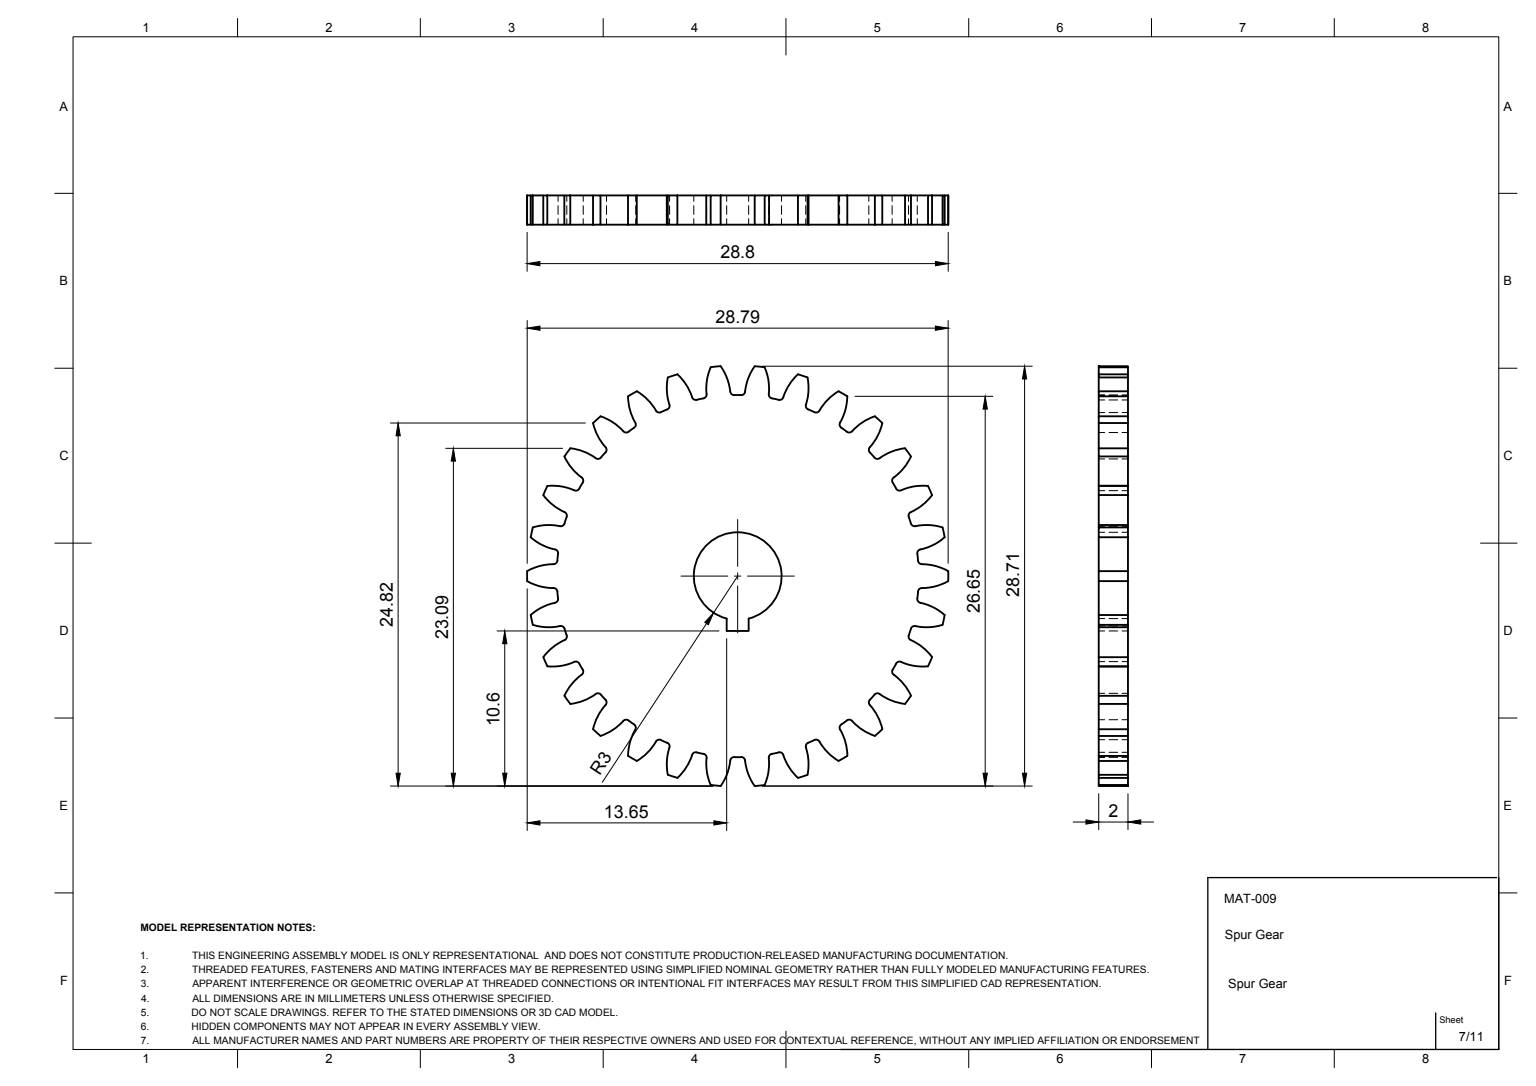
ISO-10303-21;
HEADER;
/* Generated by software containing ST-Developer
 * from STEP Tools, Inc. (www.steptools.com) 
 */

FILE_DESCRIPTION(
/* description */ ('STEP AP214'),
/* implementation_level */ '2;1');

FILE_NAME(
/* name */ 'Spur Gear.step',
/* time_stamp */ '2026-11-14T05:43:09-08:00',
/* author */ (''),
/* organization */ (''),
/* preprocessor_version */ 'ST-DEVELOPER v20.2',
/* originating_system */ 'Autodesk Translation Framework v15.17.0.0',
/* authorisation */ '');

FILE_SCHEMA (('AUTOMOTIVE_DESIGN { 1 0 10303 214 3 1 1 }'));
ENDSEC;

DATA;
#10=MECHANICAL_DESIGN_GEOMETRIC_PRESENTATION_REPRESENTATION('',(#149),#11933);
#131=SHAPE_REPRESENTATION_RELATIONSHIP('SRR','None',#11991,#140);
#140=ADVANCED_BREP_SHAPE_REPRESENTATION('',(#158),#11927);
#149=STYLED_ITEM('',(#12043),#158);
#158=MANIFOLD_SOLID_BREP('Body1',#6646);
#192=FACE_BOUND('',#825,.T.);
#193=FACE_BOUND('',#827,.T.);
#251=PLANE('',#7044);
#252=PLANE('',#7178);
#253=PLANE('',#7445);
#254=PLANE('',#7446);
#255=PLANE('',#7447);
#394=FACE_OUTER_BOUND('',#776,.T.);
#395=FACE_OUTER_BOUND('',#777,.T.);
#396=FACE_OUTER_BOUND('',#778,.T.);
#397=FACE_OUTER_BOUND('',#779,.T.);
#398=FACE_OUTER_BOUND('',#780,.T.);
#399=FACE_OUTER_BOUND('',#781,.T.);
#400=FACE_OUTER_BOUND('',#782,.T.);
#401=FACE_OUTER_BOUND('',#783,.T.);
#402=FACE_OUTER_BOUND('',#784,.T.);
#403=FACE_OUTER_BOUND('',#785,.T.);
#404=FACE_OUTER_BOUND('',#786,.T.);
#405=FACE_OUTER_BOUND('',#787,.T.);
#406=FACE_OUTER_BOUND('',#788,.T.);
#407=FACE_OUTER_BOUND('',#789,.T.);
#408=FACE_OUTER_BOUND('',#790,.T.);
#409=FACE_OUTER_BOUND('',#791,.T.);
#410=FACE_OUTER_BOUND('',#792,.T.);
#411=FACE_OUTER_BOUND('',#793,.T.);
#412=FACE_OUTER_BOUND('',#794,.T.);
#413=FACE_OUTER_BOUND('',#795,.T.);
#414=FACE_OUTER_BOUND('',#796,.T.);
#415=FACE_OUTER_BOUND('',#797,.T.);
#416=FACE_OUTER_BOUND('',#798,.T.);
#417=FACE_OUTER_BOUND('',#799,.T.);
#418=FACE_OUTER_BOUND('',#800,.T.);
#419=FACE_OUTER_BOUND('',#801,.T.);
#420=FACE_OUTER_BOUND('',#802,.T.);
#421=FACE_OUTER_BOUND('',#803,.T.);
#422=FACE_OUTER_BOUND('',#804,.T.);
#423=FACE_OUTER_BOUND('',#805,.T.);
#424=FACE_OUTER_BOUND('',#806,.T.);
#425=FACE_OUTER_BOUND('',#807,.T.);
#426=FACE_OUTER_BOUND('',#808,.T.);
#427=FACE_OUTER_BOUND('',#809,.T.);
#428=FACE_OUTER_BOUND('',#810,.T.);
#429=FACE_OUTER_BOUND('',#811,.T.);
#430=FACE_OUTER_BOUND('',#812,.T.);
#431=FACE_OUTER_BOUND('',#813,.T.);
#432=FACE_OUTER_BOUND('',#814,.T.);
#433=FACE_OUTER_BOUND('',#815,.T.);
#434=FACE_OUTER_BOUND('',#816,.T.);
#435=FACE_OUTER_BOUND('',#817,.T.);
#436=FACE_OUTER_BOUND('',#818,.T.);
#437=FACE_OUTER_BOUND('',#819,.T.);
#438=FACE_OUTER_BOUND('',#820,.T.);
#439=FACE_OUTER_BOUND('',#821,.T.);
#440=FACE_OUTER_BOUND('',#822,.T.);
#441=FACE_OUTER_BOUND('',#823,.T.);
#442=FACE_OUTER_BOUND('',#824,.T.);
#443=FACE_OUTER_BOUND('',#826,.T.);
#444=FACE_OUTER_BOUND('',#828,.T.);
#445=FACE_OUTER_BOUND('',#829,.T.);
#446=FACE_OUTER_BOUND('',#830,.T.);
#447=FACE_OUTER_BOUND('',#831,.T.);
#448=FACE_OUTER_BOUND('',#832,.T.);
#449=FACE_OUTER_BOUND('',#833,.T.);
#450=FACE_OUTER_BOUND('',#834,.T.);
#451=FACE_OUTER_BOUND('',#835,.T.);
#452=FACE_OUTER_BOUND('',#836,.T.);
#453=FACE_OUTER_BOUND('',#837,.T.);
#454=FACE_OUTER_BOUND('',#838,.T.);
#455=FACE_OUTER_BOUND('',#839,.T.);
#456=FACE_OUTER_BOUND('',#840,.T.);
#457=FACE_OUTER_BOUND('',#841,.T.);
#458=FACE_OUTER_BOUND('',#842,.T.);
#459=FACE_OUTER_BOUND('',#843,.T.);
#460=FACE_OUTER_BOUND('',#844,.T.);
#461=FACE_OUTER_BOUND('',#845,.T.);
#462=FACE_OUTER_BOUND('',#846,.T.);
#463=FACE_OUTER_BOUND('',#847,.T.);
#464=FACE_OUTER_BOUND('',#848,.T.);
#465=FACE_OUTER_BOUND('',#849,.T.);
#466=FACE_OUTER_BOUND('',#850,.T.);
#467=FACE_OUTER_BOUND('',#851,.T.);
#468=FACE_OUTER_BOUND('',#852,.T.);
#469=FACE_OUTER_BOUND('',#853,.T.);
#470=FACE_OUTER_BOUND('',#854,.T.);
#471=FACE_OUTER_BOUND('',#855,.T.);
#472=FACE_OUTER_BOUND('',#856,.T.);
#473=FACE_OUTER_BOUND('',#857,.T.);
#474=FACE_OUTER_BOUND('',#858,.T.);
#475=FACE_OUTER_BOUND('',#859,.T.);
#476=FACE_OUTER_BOUND('',#860,.T.);
#477=FACE_OUTER_BOUND('',#861,.T.);
#478=FACE_OUTER_BOUND('',#862,.T.);
#479=FACE_OUTER_BOUND('',#863,.T.);
#480=FACE_OUTER_BOUND('',#864,.T.);
#481=FACE_OUTER_BOUND('',#865,.T.);
#482=FACE_OUTER_BOUND('',#866,.T.);
#483=FACE_OUTER_BOUND('',#867,.T.);
#484=FACE_OUTER_BOUND('',#868,.T.);
#485=FACE_OUTER_BOUND('',#869,.T.);
#486=FACE_OUTER_BOUND('',#870,.T.);
#487=FACE_OUTER_BOUND('',#871,.T.);
#488=FACE_OUTER_BOUND('',#872,.T.);
#489=FACE_OUTER_BOUND('',#873,.T.);
#490=FACE_OUTER_BOUND('',#874,.T.);
#491=FACE_OUTER_BOUND('',#875,.T.);
#492=FACE_OUTER_BOUND('',#876,.T.);
#493=FACE_OUTER_BOUND('',#877,.T.);
#494=FACE_OUTER_BOUND('',#878,.T.);
#495=FACE_OUTER_BOUND('',#879,.T.);
#496=FACE_OUTER_BOUND('',#880,.T.);
#497=FACE_OUTER_BOUND('',#881,.T.);
#498=FACE_OUTER_BOUND('',#882,.T.);
#499=FACE_OUTER_BOUND('',#883,.T.);
#500=FACE_OUTER_BOUND('',#884,.T.);
#501=FACE_OUTER_BOUND('',#885,.T.);
#502=FACE_OUTER_BOUND('',#886,.T.);
#503=FACE_OUTER_BOUND('',#887,.T.);
#504=FACE_OUTER_BOUND('',#888,.T.);
#505=FACE_OUTER_BOUND('',#889,.T.);
#506=FACE_OUTER_BOUND('',#890,.T.);
#507=FACE_OUTER_BOUND('',#891,.T.);
#508=FACE_OUTER_BOUND('',#892,.T.);
#509=FACE_OUTER_BOUND('',#893,.T.);
#510=FACE_OUTER_BOUND('',#894,.T.);
#511=FACE_OUTER_BOUND('',#895,.T.);
#512=FACE_OUTER_BOUND('',#896,.T.);
#513=FACE_OUTER_BOUND('',#897,.T.);
#514=FACE_OUTER_BOUND('',#898,.T.);
#515=FACE_OUTER_BOUND('',#899,.T.);
#516=FACE_OUTER_BOUND('',#900,.T.);
#517=FACE_OUTER_BOUND('',#901,.T.);
#518=FACE_OUTER_BOUND('',#902,.T.);
#519=FACE_OUTER_BOUND('',#903,.T.);
#520=FACE_OUTER_BOUND('',#904,.T.);
#521=FACE_OUTER_BOUND('',#905,.T.);
#522=FACE_OUTER_BOUND('',#906,.T.);
#523=FACE_OUTER_BOUND('',#907,.T.);
#524=FACE_OUTER_BOUND('',#908,.T.);
#525=FACE_OUTER_BOUND('',#909,.T.);
#526=FACE_OUTER_BOUND('',#910,.T.);
#527=FACE_OUTER_BOUND('',#911,.T.);
#528=FACE_OUTER_BOUND('',#912,.T.);
#529=FACE_OUTER_BOUND('',#913,.T.);
#530=FACE_OUTER_BOUND('',#914,.T.);
#531=FACE_OUTER_BOUND('',#915,.T.);
#532=FACE_OUTER_BOUND('',#916,.T.);
#533=FACE_OUTER_BOUND('',#917,.T.);
#534=FACE_OUTER_BOUND('',#918,.T.);
#535=FACE_OUTER_BOUND('',#919,.T.);
#536=FACE_OUTER_BOUND('',#920,.T.);
#537=FACE_OUTER_BOUND('',#921,.T.);
#538=FACE_OUTER_BOUND('',#922,.T.);
#539=FACE_OUTER_BOUND('',#923,.T.);
#540=FACE_OUTER_BOUND('',#924,.T.);
#541=FACE_OUTER_BOUND('',#925,.T.);
#542=FACE_OUTER_BOUND('',#926,.T.);
#543=FACE_OUTER_BOUND('',#927,.T.);
#544=FACE_OUTER_BOUND('',#928,.T.);
#545=FACE_OUTER_BOUND('',#929,.T.);
#546=FACE_OUTER_BOUND('',#930,.T.);
#547=FACE_OUTER_BOUND('',#931,.T.);
#548=FACE_OUTER_BOUND('',#932,.T.);
#549=FACE_OUTER_BOUND('',#933,.T.);
#550=FACE_OUTER_BOUND('',#934,.T.);
#551=FACE_OUTER_BOUND('',#935,.T.);
#552=FACE_OUTER_BOUND('',#936,.T.);
#553=FACE_OUTER_BOUND('',#937,.T.);
#554=FACE_OUTER_BOUND('',#938,.T.);
#555=FACE_OUTER_BOUND('',#939,.T.);
#556=FACE_OUTER_BOUND('',#940,.T.);
#557=FACE_OUTER_BOUND('',#941,.T.);
#558=FACE_OUTER_BOUND('',#942,.T.);
#559=FACE_OUTER_BOUND('',#943,.T.);
#560=FACE_OUTER_BOUND('',#944,.T.);
#561=FACE_OUTER_BOUND('',#945,.T.);
#562=FACE_OUTER_BOUND('',#946,.T.);
#563=FACE_OUTER_BOUND('',#947,.T.);
#564=FACE_OUTER_BOUND('',#948,.T.);
#565=FACE_OUTER_BOUND('',#949,.T.);
#566=FACE_OUTER_BOUND('',#950,.T.);
#567=FACE_OUTER_BOUND('',#951,.T.);
#568=FACE_OUTER_BOUND('',#952,.T.);
#569=FACE_OUTER_BOUND('',#953,.T.);
#570=FACE_OUTER_BOUND('',#954,.T.);
#571=FACE_OUTER_BOUND('',#955,.T.);
#572=FACE_OUTER_BOUND('',#956,.T.);
#573=FACE_OUTER_BOUND('',#957,.T.);
#574=FACE_OUTER_BOUND('',#958,.T.);
#575=FACE_OUTER_BOUND('',#959,.T.);
#576=FACE_OUTER_BOUND('',#960,.T.);
#577=FACE_OUTER_BOUND('',#961,.T.);
#578=FACE_OUTER_BOUND('',#962,.T.);
#579=FACE_OUTER_BOUND('',#963,.T.);
#776=EDGE_LOOP('',(#4486,#4487,#4488,#4489));
#777=EDGE_LOOP('',(#4490,#4491,#4492,#4493));
#778=EDGE_LOOP('',(#4494,#4495,#4496,#4497));
#779=EDGE_LOOP('',(#4498,#4499,#4500,#4501));
#780=EDGE_LOOP('',(#4502,#4503,#4504,#4505));
#781=EDGE_LOOP('',(#4506,#4507,#4508,#4509));
#782=EDGE_LOOP('',(#4510,#4511,#4512,#4513));
#783=EDGE_LOOP('',(#4514,#4515,#4516,#4517));
#784=EDGE_LOOP('',(#4518,#4519,#4520,#4521));
#785=EDGE_LOOP('',(#4522,#4523,#4524,#4525));
#786=EDGE_LOOP('',(#4526,#4527,#4528,#4529));
#787=EDGE_LOOP('',(#4530,#4531,#4532,#4533));
#788=EDGE_LOOP('',(#4534,#4535,#4536,#4537));
#789=EDGE_LOOP('',(#4538,#4539,#4540,#4541));
#790=EDGE_LOOP('',(#4542,#4543,#4544,#4545));
#791=EDGE_LOOP('',(#4546,#4547,#4548,#4549));
#792=EDGE_LOOP('',(#4550,#4551,#4552,#4553));
#793=EDGE_LOOP('',(#4554,#4555,#4556,#4557));
#794=EDGE_LOOP('',(#4558,#4559,#4560,#4561));
#795=EDGE_LOOP('',(#4562,#4563,#4564,#4565));
#796=EDGE_LOOP('',(#4566,#4567,#4568,#4569));
#797=EDGE_LOOP('',(#4570,#4571,#4572,#4573));
#798=EDGE_LOOP('',(#4574,#4575,#4576,#4577));
#799=EDGE_LOOP('',(#4578,#4579,#4580,#4581));
#800=EDGE_LOOP('',(#4582,#4583,#4584,#4585));
#801=EDGE_LOOP('',(#4586,#4587,#4588,#4589));
#802=EDGE_LOOP('',(#4590,#4591,#4592,#4593));
#803=EDGE_LOOP('',(#4594,#4595,#4596,#4597));
#804=EDGE_LOOP('',(#4598,#4599,#4600,#4601));
#805=EDGE_LOOP('',(#4602,#4603,#4604,#4605));
#806=EDGE_LOOP('',(#4606,#4607,#4608,#4609));
#807=EDGE_LOOP('',(#4610,#4611,#4612,#4613));
#808=EDGE_LOOP('',(#4614,#4615,#4616,#4617));
#809=EDGE_LOOP('',(#4618,#4619,#4620,#4621));
#810=EDGE_LOOP('',(#4622,#4623,#4624,#4625));
#811=EDGE_LOOP('',(#4626,#4627,#4628,#4629));
#812=EDGE_LOOP('',(#4630,#4631,#4632,#4633));
#813=EDGE_LOOP('',(#4634,#4635,#4636,#4637));
#814=EDGE_LOOP('',(#4638,#4639,#4640,#4641));
#815=EDGE_LOOP('',(#4642,#4643,#4644,#4645));
#816=EDGE_LOOP('',(#4646,#4647,#4648,#4649));
#817=EDGE_LOOP('',(#4650,#4651,#4652,#4653));
#818=EDGE_LOOP('',(#4654,#4655,#4656,#4657));
#819=EDGE_LOOP('',(#4658,#4659,#4660,#4661));
#820=EDGE_LOOP('',(#4662,#4663,#4664,#4665));
#821=EDGE_LOOP('',(#4666,#4667,#4668,#4669));
#822=EDGE_LOOP('',(#4670,#4671,#4672,#4673));
#823=EDGE_LOOP('',(#4674,#4675,#4676,#4677));
#824=EDGE_LOOP('',(#4678,#4679,#4680,#4681,#4682,#4683,#4684,#4685,#4686,
#4687,#4688,#4689,#4690,#4691,#4692,#4693,#4694,#4695,#4696,#4697,#4698,
#4699,#4700,#4701,#4702,#4703,#4704,#4705,#4706,#4707,#4708,#4709,#4710,
#4711,#4712,#4713,#4714,#4715,#4716,#4717,#4718,#4719,#4720,#4721,#4722,
#4723,#4724,#4725,#4726,#4727,#4728,#4729,#4730,#4731,#4732,#4733,#4734,
#4735,#4736,#4737,#4738,#4739,#4740,#4741,#4742,#4743,#4744,#4745,#4746,
#4747,#4748,#4749,#4750,#4751,#4752,#4753,#4754,#4755,#4756,#4757,#4758,
#4759,#4760,#4761,#4762,#4763,#4764,#4765,#4766,#4767,#4768,#4769,#4770,
#4771,#4772,#4773,#4774,#4775,#4776,#4777,#4778,#4779,#4780,#4781,#4782,
#4783,#4784,#4785,#4786,#4787,#4788,#4789,#4790,#4791,#4792,#4793,#4794,
#4795,#4796,#4797,#4798,#4799,#4800,#4801,#4802,#4803,#4804,#4805,#4806,
#4807,#4808,#4809,#4810,#4811,#4812,#4813,#4814,#4815,#4816,#4817,#4818,
#4819,#4820,#4821,#4822,#4823,#4824,#4825,#4826,#4827,#4828,#4829,#4830,
#4831,#4832,#4833,#4834,#4835,#4836,#4837,#4838,#4839,#4840,#4841,#4842,
#4843,#4844,#4845,#4846,#4847,#4848,#4849,#4850,#4851,#4852,#4853,#4854,
#4855,#4856,#4857));
#825=EDGE_LOOP('',(#4858,#4859,#4860,#4861));
#826=EDGE_LOOP('',(#4862,#4863,#4864,#4865,#4866,#4867,#4868,#4869,#4870,
#4871,#4872,#4873,#4874,#4875,#4876,#4877,#4878,#4879,#4880,#4881,#4882,
#4883,#4884,#4885,#4886,#4887,#4888,#4889,#4890,#4891,#4892,#4893,#4894,
#4895,#4896,#4897,#4898,#4899,#4900,#4901,#4902,#4903,#4904,#4905,#4906,
#4907,#4908,#4909,#4910,#4911,#4912,#4913,#4914,#4915,#4916,#4917,#4918,
#4919,#4920,#4921,#4922,#4923,#4924,#4925,#4926,#4927,#4928,#4929,#4930,
#4931,#4932,#4933,#4934,#4935,#4936,#4937,#4938,#4939,#4940,#4941,#4942,
#4943,#4944,#4945,#4946,#4947,#4948,#4949,#4950,#4951,#4952,#4953,#4954,
#4955,#4956,#4957,#4958,#4959,#4960,#4961,#4962,#4963,#4964,#4965,#4966,
#4967,#4968,#4969,#4970,#4971,#4972,#4973,#4974,#4975,#4976,#4977,#4978,
#4979,#4980,#4981,#4982,#4983,#4984,#4985,#4986,#4987,#4988,#4989,#4990,
#4991,#4992,#4993,#4994,#4995,#4996,#4997,#4998,#4999,#5000,#5001,#5002,
#5003,#5004,#5005,#5006,#5007,#5008,#5009,#5010,#5011,#5012,#5013,#5014,
#5015,#5016,#5017,#5018,#5019,#5020,#5021,#5022,#5023,#5024,#5025,#5026,
#5027,#5028,#5029,#5030,#5031,#5032,#5033,#5034,#5035,#5036,#5037,#5038,
#5039,#5040,#5041));
#827=EDGE_LOOP('',(#5042,#5043,#5044,#5045));
#828=EDGE_LOOP('',(#5046,#5047,#5048,#5049));
#829=EDGE_LOOP('',(#5050,#5051,#5052,#5053));
#830=EDGE_LOOP('',(#5054,#5055,#5056,#5057));
#831=EDGE_LOOP('',(#5058,#5059,#5060,#5061));
#832=EDGE_LOOP('',(#5062,#5063,#5064,#5065));
#833=EDGE_LOOP('',(#5066,#5067,#5068,#5069));
#834=EDGE_LOOP('',(#5070,#5071,#5072,#5073));
#835=EDGE_LOOP('',(#5074,#5075,#5076,#5077));
#836=EDGE_LOOP('',(#5078,#5079,#5080,#5081));
#837=EDGE_LOOP('',(#5082,#5083,#5084,#5085));
#838=EDGE_LOOP('',(#5086,#5087,#5088,#5089));
#839=EDGE_LOOP('',(#5090,#5091,#5092,#5093));
#840=EDGE_LOOP('',(#5094,#5095,#5096,#5097));
#841=EDGE_LOOP('',(#5098,#5099,#5100,#5101));
#842=EDGE_LOOP('',(#5102,#5103,#5104,#5105));
#843=EDGE_LOOP('',(#5106,#5107,#5108,#5109));
#844=EDGE_LOOP('',(#5110,#5111,#5112,#5113));
#845=EDGE_LOOP('',(#5114,#5115,#5116,#5117));
#846=EDGE_LOOP('',(#5118,#5119,#5120,#5121));
#847=EDGE_LOOP('',(#5122,#5123,#5124,#5125));
#848=EDGE_LOOP('',(#5126,#5127,#5128,#5129));
#849=EDGE_LOOP('',(#5130,#5131,#5132,#5133));
#850=EDGE_LOOP('',(#5134,#5135,#5136,#5137));
#851=EDGE_LOOP('',(#5138,#5139,#5140,#5141));
#852=EDGE_LOOP('',(#5142,#5143,#5144,#5145));
#853=EDGE_LOOP('',(#5146,#5147,#5148,#5149));
#854=EDGE_LOOP('',(#5150,#5151,#5152,#5153));
#855=EDGE_LOOP('',(#5154,#5155,#5156,#5157));
#856=EDGE_LOOP('',(#5158,#5159,#5160,#5161));
#857=EDGE_LOOP('',(#5162,#5163,#5164,#5165));
#858=EDGE_LOOP('',(#5166,#5167,#5168,#5169));
#859=EDGE_LOOP('',(#5170,#5171,#5172,#5173));
#860=EDGE_LOOP('',(#5174,#5175,#5176,#5177));
#861=EDGE_LOOP('',(#5178,#5179,#5180,#5181));
#862=EDGE_LOOP('',(#5182,#5183,#5184,#5185));
#863=EDGE_LOOP('',(#5186,#5187,#5188,#5189));
#864=EDGE_LOOP('',(#5190,#5191,#5192,#5193));
#865=EDGE_LOOP('',(#5194,#5195,#5196,#5197));
#866=EDGE_LOOP('',(#5198,#5199,#5200,#5201));
#867=EDGE_LOOP('',(#5202,#5203,#5204,#5205));
#868=EDGE_LOOP('',(#5206,#5207,#5208,#5209));
#869=EDGE_LOOP('',(#5210,#5211,#5212,#5213));
#870=EDGE_LOOP('',(#5214,#5215,#5216,#5217));
#871=EDGE_LOOP('',(#5218,#5219,#5220,#5221));
#872=EDGE_LOOP('',(#5222,#5223,#5224,#5225));
#873=EDGE_LOOP('',(#5226,#5227,#5228,#5229));
#874=EDGE_LOOP('',(#5230,#5231,#5232,#5233));
#875=EDGE_LOOP('',(#5234,#5235,#5236,#5237));
#876=EDGE_LOOP('',(#5238,#5239,#5240,#5241));
#877=EDGE_LOOP('',(#5242,#5243,#5244,#5245));
#878=EDGE_LOOP('',(#5246,#5247,#5248,#5249));
#879=EDGE_LOOP('',(#5250,#5251,#5252,#5253));
#880=EDGE_LOOP('',(#5254,#5255,#5256,#5257));
#881=EDGE_LOOP('',(#5258,#5259,#5260,#5261));
#882=EDGE_LOOP('',(#5262,#5263,#5264,#5265));
#883=EDGE_LOOP('',(#5266,#5267,#5268,#5269));
#884=EDGE_LOOP('',(#5270,#5271,#5272,#5273));
#885=EDGE_LOOP('',(#5274,#5275,#5276,#5277));
#886=EDGE_LOOP('',(#5278,#5279,#5280,#5281));
#887=EDGE_LOOP('',(#5282,#5283,#5284,#5285));
#888=EDGE_LOOP('',(#5286,#5287,#5288,#5289));
#889=EDGE_LOOP('',(#5290,#5291,#5292,#5293));
#890=EDGE_LOOP('',(#5294,#5295,#5296,#5297));
#891=EDGE_LOOP('',(#5298,#5299,#5300,#5301));
#892=EDGE_LOOP('',(#5302,#5303,#5304,#5305));
#893=EDGE_LOOP('',(#5306,#5307,#5308,#5309));
#894=EDGE_LOOP('',(#5310,#5311,#5312,#5313));
#895=EDGE_LOOP('',(#5314,#5315,#5316,#5317));
#896=EDGE_LOOP('',(#5318,#5319,#5320,#5321));
#897=EDGE_LOOP('',(#5322,#5323,#5324,#5325));
#898=EDGE_LOOP('',(#5326,#5327,#5328,#5329));
#899=EDGE_LOOP('',(#5330,#5331,#5332,#5333));
#900=EDGE_LOOP('',(#5334,#5335,#5336,#5337));
#901=EDGE_LOOP('',(#5338,#5339,#5340,#5341));
#902=EDGE_LOOP('',(#5342,#5343,#5344,#5345));
#903=EDGE_LOOP('',(#5346,#5347,#5348,#5349));
#904=EDGE_LOOP('',(#5350,#5351,#5352,#5353));
#905=EDGE_LOOP('',(#5354,#5355,#5356,#5357));
#906=EDGE_LOOP('',(#5358,#5359,#5360,#5361));
#907=EDGE_LOOP('',(#5362,#5363,#5364,#5365));
#908=EDGE_LOOP('',(#5366,#5367,#5368,#5369));
#909=EDGE_LOOP('',(#5370,#5371,#5372,#5373));
#910=EDGE_LOOP('',(#5374,#5375,#5376,#5377));
#911=EDGE_LOOP('',(#5378,#5379,#5380,#5381));
#912=EDGE_LOOP('',(#5382,#5383,#5384,#5385));
#913=EDGE_LOOP('',(#5386,#5387,#5388,#5389));
#914=EDGE_LOOP('',(#5390,#5391,#5392,#5393));
#915=EDGE_LOOP('',(#5394,#5395,#5396,#5397));
#916=EDGE_LOOP('',(#5398,#5399,#5400,#5401));
#917=EDGE_LOOP('',(#5402,#5403,#5404,#5405));
#918=EDGE_LOOP('',(#5406,#5407,#5408,#5409));
#919=EDGE_LOOP('',(#5410,#5411,#5412,#5413));
#920=EDGE_LOOP('',(#5414,#5415,#5416,#5417));
#921=EDGE_LOOP('',(#5418,#5419,#5420,#5421));
#922=EDGE_LOOP('',(#5422,#5423,#5424,#5425));
#923=EDGE_LOOP('',(#5426,#5427,#5428,#5429));
#924=EDGE_LOOP('',(#5430,#5431,#5432,#5433));
#925=EDGE_LOOP('',(#5434,#5435,#5436,#5437));
#926=EDGE_LOOP('',(#5438,#5439,#5440,#5441));
#927=EDGE_LOOP('',(#5442,#5443,#5444,#5445));
#928=EDGE_LOOP('',(#5446,#5447,#5448,#5449));
#929=EDGE_LOOP('',(#5450,#5451,#5452,#5453));
#930=EDGE_LOOP('',(#5454,#5455,#5456,#5457));
#931=EDGE_LOOP('',(#5458,#5459,#5460,#5461));
#932=EDGE_LOOP('',(#5462,#5463,#5464,#5465));
#933=EDGE_LOOP('',(#5466,#5467,#5468,#5469));
#934=EDGE_LOOP('',(#5470,#5471,#5472,#5473));
#935=EDGE_LOOP('',(#5474,#5475,#5476,#5477));
#936=EDGE_LOOP('',(#5478,#5479,#5480,#5481));
#937=EDGE_LOOP('',(#5482,#5483,#5484,#5485));
#938=EDGE_LOOP('',(#5486,#5487,#5488,#5489));
#939=EDGE_LOOP('',(#5490,#5491,#5492,#5493));
#940=EDGE_LOOP('',(#5494,#5495,#5496,#5497));
#941=EDGE_LOOP('',(#5498,#5499,#5500,#5501));
#942=EDGE_LOOP('',(#5502,#5503,#5504,#5505));
#943=EDGE_LOOP('',(#5506,#5507,#5508,#5509));
#944=EDGE_LOOP('',(#5510,#5511,#5512,#5513));
#945=EDGE_LOOP('',(#5514,#5515,#5516,#5517));
#946=EDGE_LOOP('',(#5518,#5519,#5520,#5521));
#947=EDGE_LOOP('',(#5522,#5523,#5524,#5525));
#948=EDGE_LOOP('',(#5526,#5527,#5528,#5529));
#949=EDGE_LOOP('',(#5530,#5531,#5532,#5533));
#950=EDGE_LOOP('',(#5534,#5535,#5536,#5537));
#951=EDGE_LOOP('',(#5538,#5539,#5540,#5541));
#952=EDGE_LOOP('',(#5542,#5543,#5544,#5545));
#953=EDGE_LOOP('',(#5546,#5547,#5548,#5549));
#954=EDGE_LOOP('',(#5550,#5551,#5552,#5553));
#955=EDGE_LOOP('',(#5554,#5555,#5556,#5557));
#956=EDGE_LOOP('',(#5558,#5559,#5560,#5561));
#957=EDGE_LOOP('',(#5562,#5563,#5564,#5565));
#958=EDGE_LOOP('',(#5566,#5567,#5568,#5569));
#959=EDGE_LOOP('',(#5570,#5571,#5572,#5573));
#960=EDGE_LOOP('',(#5574,#5575,#5576,#5577));
#961=EDGE_LOOP('',(#5578,#5579,#5580,#5581));
#962=EDGE_LOOP('',(#5582,#5583,#5584,#5585));
#963=EDGE_LOOP('',(#5586,#5587,#5588,#5589));
#1191=LINE('',#10304,#1653);
#1192=LINE('',#10307,#1654);
#1193=LINE('',#10313,#1655);
#1194=LINE('',#10316,#1656);
#1195=LINE('',#10321,#1657);
#1196=LINE('',#10328,#1658);
#1197=LINE('',#10331,#1659);
#1198=LINE('',#10336,#1660);
#1199=LINE('',#10343,#1661);
#1200=LINE('',#10346,#1662);
#1201=LINE('',#10352,#1663);
#1202=LINE('',#10358,#1664);
#1203=LINE('',#10361,#1665);
#1204=LINE('',#10367,#1666);
#1205=LINE('',#10373,#1667);
#1206=LINE('',#10376,#1668);
#1207=LINE('',#10382,#1669);
#1208=LINE('',#10385,#1670);
#1209=LINE('',#10391,#1671);
#1210=LINE('',#10394,#1672);
#1211=LINE('',#10400,#1673);
#1212=LINE('',#10403,#1674);
#1213=LINE('',#10409,#1675);
#1214=LINE('',#10412,#1676);
#1215=LINE('',#10418,#1677);
#1216=LINE('',#10421,#1678);
#1217=LINE('',#10427,#1679);
#1218=LINE('',#10430,#1680);
#1219=LINE('',#10436,#1681);
#1220=LINE('',#10439,#1682);
#1221=LINE('',#10445,#1683);
#1222=LINE('',#10448,#1684);
#1223=LINE('',#10454,#1685);
#1224=LINE('',#10457,#1686);
#1225=LINE('',#10463,#1687);
#1226=LINE('',#10466,#1688);
#1227=LINE('',#10472,#1689);
#1228=LINE('',#10475,#1690);
#1229=LINE('',#10481,#1691);
#1230=LINE('',#10484,#1692);
#1231=LINE('',#10490,#1693);
#1232=LINE('',#10493,#1694);
#1233=LINE('',#10499,#1695);
#1234=LINE('',#10502,#1696);
#1235=LINE('',#10508,#1697);
#1236=LINE('',#10511,#1698);
#1237=LINE('',#10517,#1699);
#1238=LINE('',#10520,#1700);
#1239=LINE('',#10526,#1701);
#1240=LINE('',#10529,#1702);
#1241=LINE('',#10535,#1703);
#1242=LINE('',#10538,#1704);
#1243=LINE('',#10544,#1705);
#1244=LINE('',#10547,#1706);
#1245=LINE('',#10553,#1707);
#1246=LINE('',#10556,#1708);
#1247=LINE('',#10562,#1709);
#1248=LINE('',#10565,#1710);
#1249=LINE('',#10571,#1711);
#1250=LINE('',#10574,#1712);
#1251=LINE('',#10580,#1713);
#1252=LINE('',#10583,#1714);
#1253=LINE('',#10588,#1715);
#1254=LINE('',#10594,#1716);
#1255=LINE('',#10600,#1717);
#1256=LINE('',#10607,#1718);
#1257=LINE('',#10610,#1719);
#1258=LINE('',#10616,#1720);
#1259=LINE('',#10619,#1721);
#1260=LINE('',#10625,#1722);
#1261=LINE('',#10628,#1723);
#1262=LINE('',#10634,#1724);
#1263=LINE('',#10637,#1725);
#1264=LINE('',#10643,#1726);
#1265=LINE('',#10646,#1727);
#1266=LINE('',#10652,#1728);
#1267=LINE('',#10655,#1729);
#1268=LINE('',#10661,#1730);
#1269=LINE('',#10664,#1731);
#1270=LINE('',#10670,#1732);
#1271=LINE('',#10673,#1733);
#1272=LINE('',#10679,#1734);
#1273=LINE('',#10682,#1735);
#1274=LINE('',#10688,#1736);
#1275=LINE('',#10691,#1737);
#1276=LINE('',#10697,#1738);
#1277=LINE('',#10700,#1739);
#1278=LINE('',#10706,#1740);
#1279=LINE('',#10709,#1741);
#1280=LINE('',#10938,#1742);
#1281=LINE('',#10940,#1743);
#1282=LINE('',#10941,#1744);
#1283=LINE('',#11170,#1745);
#1284=LINE('',#11172,#1746);
#1285=LINE('',#11173,#1747);
#1286=LINE('',#11175,#1748);
#1287=LINE('',#11177,#1749);
#1288=LINE('',#11179,#1750);
#1289=LINE('',#11181,#1751);
#1290=LINE('',#11182,#1752);
#1291=LINE('',#11186,#1753);
#1292=LINE('',#11188,#1754);
#1293=LINE('',#11190,#1755);
#1294=LINE('',#11192,#1756);
#1295=LINE('',#11196,#1757);
#1296=LINE('',#11198,#1758);
#1297=LINE('',#11202,#1759);
#1298=LINE('',#11204,#1760);
#1299=LINE('',#11208,#1761);
#1300=LINE('',#11210,#1762);
#1301=LINE('',#11214,#1763);
#1302=LINE('',#11216,#1764);
#1303=LINE('',#11220,#1765);
#1304=LINE('',#11222,#1766);
#1305=LINE('',#11225,#1767);
#1306=LINE('',#11228,#1768);
#1307=LINE('',#11231,#1769);
#1308=LINE('',#11234,#1770);
#1309=LINE('',#11237,#1771);
#1310=LINE('',#11240,#1772);
#1311=LINE('',#11243,#1773);
#1312=LINE('',#11246,#1774);
#1313=LINE('',#11249,#1775);
#1314=LINE('',#11252,#1776);
#1315=LINE('',#11255,#1777);
#1316=LINE('',#11257,#1778);
#1317=LINE('',#11260,#1779);
#1318=LINE('',#11262,#1780);
#1319=LINE('',#11265,#1781);
#1320=LINE('',#11267,#1782);
#1321=LINE('',#11270,#1783);
#1322=LINE('',#11272,#1784);
#1323=LINE('',#11275,#1785);
#1324=LINE('',#11277,#1786);
#1325=LINE('',#11279,#1787);
#1326=LINE('',#11281,#1788);
#1327=LINE('',#11284,#1789);
#1328=LINE('',#11286,#1790);
#1329=LINE('',#11288,#1791);
#1330=LINE('',#11290,#1792);
#1331=LINE('',#11293,#1793);
#1332=LINE('',#11295,#1794);
#1333=LINE('',#11297,#1795);
#1334=LINE('',#11299,#1796);
#1335=LINE('',#11302,#1797);
#1336=LINE('',#11304,#1798);
#1337=LINE('',#11306,#1799);
#1338=LINE('',#11308,#1800);
#1339=LINE('',#11311,#1801);
#1340=LINE('',#11313,#1802);
#1341=LINE('',#11315,#1803);
#1342=LINE('',#11317,#1804);
#1343=LINE('',#11320,#1805);
#1344=LINE('',#11322,#1806);
#1345=LINE('',#11324,#1807);
#1346=LINE('',#11326,#1808);
#1347=LINE('',#11329,#1809);
#1348=LINE('',#11331,#1810);
#1349=LINE('',#11333,#1811);
#1350=LINE('',#11335,#1812);
#1351=LINE('',#11338,#1813);
#1352=LINE('',#11340,#1814);
#1353=LINE('',#11342,#1815);
#1354=LINE('',#11344,#1816);
#1355=LINE('',#11347,#1817);
#1356=LINE('',#11349,#1818);
#1357=LINE('',#11351,#1819);
#1358=LINE('',#11353,#1820);
#1359=LINE('',#11356,#1821);
#1360=LINE('',#11358,#1822);
#1361=LINE('',#11360,#1823);
#1362=LINE('',#11362,#1824);
#1363=LINE('',#11365,#1825);
#1364=LINE('',#11367,#1826);
#1365=LINE('',#11369,#1827);
#1366=LINE('',#11371,#1828);
#1367=LINE('',#11374,#1829);
#1368=LINE('',#11376,#1830);
#1369=LINE('',#11378,#1831);
#1370=LINE('',#11380,#1832);
#1371=LINE('',#11383,#1833);
#1372=LINE('',#11385,#1834);
#1373=LINE('',#11387,#1835);
#1374=LINE('',#11389,#1836);
#1375=LINE('',#11392,#1837);
#1376=LINE('',#11394,#1838);
#1377=LINE('',#11396,#1839);
#1378=LINE('',#11398,#1840);
#1379=LINE('',#11401,#1841);
#1380=LINE('',#11403,#1842);
#1653=VECTOR('',#8069,1000.);
#1654=VECTOR('',#8072,1000.);
#1655=VECTOR('',#8077,1000.);
#1656=VECTOR('',#8080,1000.);
#1657=VECTOR('',#8085,1000.);
#1658=VECTOR('',#8092,1000.);
#1659=VECTOR('',#8095,1000.);
#1660=VECTOR('',#8100,1000.);
#1661=VECTOR('',#8107,1000.);
#1662=VECTOR('',#8110,1000.);
#1663=VECTOR('',#8117,1000.);
#1664=VECTOR('',#8122,1000.);
#1665=VECTOR('',#8125,1000.);
#1666=VECTOR('',#8132,1000.);
#1667=VECTOR('',#8137,1000.);
#1668=VECTOR('',#8140,1000.);
#1669=VECTOR('',#8145,1000.);
#1670=VECTOR('',#8148,1000.);
#1671=VECTOR('',#8153,1000.);
#1672=VECTOR('',#8156,1000.);
#1673=VECTOR('',#8161,1000.);
#1674=VECTOR('',#8164,1000.);
#1675=VECTOR('',#8169,1000.);
#1676=VECTOR('',#8172,1000.);
#1677=VECTOR('',#8177,1000.);
#1678=VECTOR('',#8180,1000.);
#1679=VECTOR('',#8185,1000.);
#1680=VECTOR('',#8188,1000.);
#1681=VECTOR('',#8193,1000.);
#1682=VECTOR('',#8196,1000.);
#1683=VECTOR('',#8201,1000.);
#1684=VECTOR('',#8204,1000.);
#1685=VECTOR('',#8209,1000.);
#1686=VECTOR('',#8212,1000.);
#1687=VECTOR('',#8217,1000.);
#1688=VECTOR('',#8220,1000.);
#1689=VECTOR('',#8225,1000.);
#1690=VECTOR('',#8228,1000.);
#1691=VECTOR('',#8233,1000.);
#1692=VECTOR('',#8236,1000.);
#1693=VECTOR('',#8241,1000.);
#1694=VECTOR('',#8244,1000.);
#1695=VECTOR('',#8249,1000.);
#1696=VECTOR('',#8252,1000.);
#1697=VECTOR('',#8257,1000.);
#1698=VECTOR('',#8260,1000.);
#1699=VECTOR('',#8265,1000.);
#1700=VECTOR('',#8268,1000.);
#1701=VECTOR('',#8273,1000.);
#1702=VECTOR('',#8276,1000.);
#1703=VECTOR('',#8281,1000.);
#1704=VECTOR('',#8284,1000.);
#1705=VECTOR('',#8289,1000.);
#1706=VECTOR('',#8292,1000.);
#1707=VECTOR('',#8297,1000.);
#1708=VECTOR('',#8300,1000.);
#1709=VECTOR('',#8305,1000.);
#1710=VECTOR('',#8308,1000.);
#1711=VECTOR('',#8313,1000.);
#1712=VECTOR('',#8316,1000.);
#1713=VECTOR('',#8321,1000.);
#1714=VECTOR('',#8324,1000.);
#1715=VECTOR('',#8329,1000.);
#1716=VECTOR('',#8336,1000.);
#1717=VECTOR('',#8343,1000.);
#1718=VECTOR('',#8350,1000.);
#1719=VECTOR('',#8353,1000.);
#1720=VECTOR('',#8358,1000.);
#1721=VECTOR('',#8361,1000.);
#1722=VECTOR('',#8366,1000.);
#1723=VECTOR('',#8369,1000.);
#1724=VECTOR('',#8374,1000.);
#1725=VECTOR('',#8377,1000.);
#1726=VECTOR('',#8382,1000.);
#1727=VECTOR('',#8385,1000.);
#1728=VECTOR('',#8390,1000.);
#1729=VECTOR('',#8393,1000.);
#1730=VECTOR('',#8398,1000.);
#1731=VECTOR('',#8401,1000.);
#1732=VECTOR('',#8406,1000.);
#1733=VECTOR('',#8409,1000.);
#1734=VECTOR('',#8414,1000.);
#1735=VECTOR('',#8417,1000.);
#1736=VECTOR('',#8422,1000.);
#1737=VECTOR('',#8425,1000.);
#1738=VECTOR('',#8430,1000.);
#1739=VECTOR('',#8433,1000.);
#1740=VECTOR('',#8438,1000.);
#1741=VECTOR('',#8441,1000.);
#1742=VECTOR('',#8710,1000.);
#1743=VECTOR('',#8711,1000.);
#1744=VECTOR('',#8712,1000.);
#1745=VECTOR('',#8981,1000.);
#1746=VECTOR('',#8982,1000.);
#1747=VECTOR('',#8983,1000.);
#1748=VECTOR('',#8986,1000.);
#1749=VECTOR('',#8989,1000.);
#1750=VECTOR('',#8992,1000.);
#1751=VECTOR('',#8995,1000.);
#1752=VECTOR('',#8996,1000.);
#1753=VECTOR('',#9003,1000.);
#1754=VECTOR('',#9006,1000.);
#1755=VECTOR('',#9009,1000.);
#1756=VECTOR('',#9012,1000.);
#1757=VECTOR('',#9019,1000.);
#1758=VECTOR('',#9022,1000.);
#1759=VECTOR('',#9029,1000.);
#1760=VECTOR('',#9032,1000.);
#1761=VECTOR('',#9039,1000.);
#1762=VECTOR('',#9042,1000.);
#1763=VECTOR('',#9049,1000.);
#1764=VECTOR('',#9052,1000.);
#1765=VECTOR('',#9059,1000.);
#1766=VECTOR('',#9062,1000.);
#1767=VECTOR('',#9067,1000.);
#1768=VECTOR('',#9072,1000.);
#1769=VECTOR('',#9077,1000.);
#1770=VECTOR('',#9082,1000.);
#1771=VECTOR('',#9087,1000.);
#1772=VECTOR('',#9092,1000.);
#1773=VECTOR('',#9097,1000.);
#1774=VECTOR('',#9102,1000.);
#1775=VECTOR('',#9107,1000.);
#1776=VECTOR('',#9112,1000.);
#1777=VECTOR('',#9117,1000.);
#1778=VECTOR('',#9120,1000.);
#1779=VECTOR('',#9125,1000.);
#1780=VECTOR('',#9128,1000.);
#1781=VECTOR('',#9133,1000.);
#1782=VECTOR('',#9136,1000.);
#1783=VECTOR('',#9141,1000.);
#1784=VECTOR('',#9144,1000.);
#1785=VECTOR('',#9149,1000.);
#1786=VECTOR('',#9152,1000.);
#1787=VECTOR('',#9155,1000.);
#1788=VECTOR('',#9158,1000.);
#1789=VECTOR('',#9163,1000.);
#1790=VECTOR('',#9166,1000.);
#1791=VECTOR('',#9169,1000.);
#1792=VECTOR('',#9172,1000.);
#1793=VECTOR('',#9177,1000.);
#1794=VECTOR('',#9180,1000.);
#1795=VECTOR('',#9183,1000.);
#1796=VECTOR('',#9186,1000.);
#1797=VECTOR('',#9191,1000.);
#1798=VECTOR('',#9194,1000.);
#1799=VECTOR('',#9197,1000.);
#1800=VECTOR('',#9200,1000.);
#1801=VECTOR('',#9205,1000.);
#1802=VECTOR('',#9208,1000.);
#1803=VECTOR('',#9211,1000.);
#1804=VECTOR('',#9214,1000.);
#1805=VECTOR('',#9219,1000.);
#1806=VECTOR('',#9222,1000.);
#1807=VECTOR('',#9225,1000.);
#1808=VECTOR('',#9228,1000.);
#1809=VECTOR('',#9233,1000.);
#1810=VECTOR('',#9236,1000.);
#1811=VECTOR('',#9239,1000.);
#1812=VECTOR('',#9242,1000.);
#1813=VECTOR('',#9247,1000.);
#1814=VECTOR('',#9250,1000.);
#1815=VECTOR('',#9253,1000.);
#1816=VECTOR('',#9256,1000.);
#1817=VECTOR('',#9261,1000.);
#1818=VECTOR('',#9264,1000.);
#1819=VECTOR('',#9267,1000.);
#1820=VECTOR('',#9270,1000.);
#1821=VECTOR('',#9275,1000.);
#1822=VECTOR('',#9278,1000.);
#1823=VECTOR('',#9281,1000.);
#1824=VECTOR('',#9284,1000.);
#1825=VECTOR('',#9289,1000.);
#1826=VECTOR('',#9292,1000.);
#1827=VECTOR('',#9295,1000.);
#1828=VECTOR('',#9298,1000.);
#1829=VECTOR('',#9303,1000.);
#1830=VECTOR('',#9306,1000.);
#1831=VECTOR('',#9309,1000.);
#1832=VECTOR('',#9312,1000.);
#1833=VECTOR('',#9317,1000.);
#1834=VECTOR('',#9320,1000.);
#1835=VECTOR('',#9323,1000.);
#1836=VECTOR('',#9326,1000.);
#1837=VECTOR('',#9331,1000.);
#1838=VECTOR('',#9334,1000.);
#1839=VECTOR('',#9337,1000.);
#1840=VECTOR('',#9340,1000.);
#1841=VECTOR('',#9345,1000.);
#1842=VECTOR('',#9348,1000.);
#2064=CIRCLE('',#6901,3.);
#2065=CIRCLE('',#6902,3.);
#2066=CIRCLE('',#6904,0.269999999999999);
#2067=CIRCLE('',#6905,0.269999999999999);
#2068=CIRCLE('',#6907,3.68751484013274);
#2069=CIRCLE('',#6908,3.68751484013273);
#2070=CIRCLE('',#6910,0.269999999999999);
#2071=CIRCLE('',#6911,0.269999999999999);
#2072=CIRCLE('',#6913,3.68751484013275);
#2073=CIRCLE('',#6914,3.68751484013275);
#2074=CIRCLE('',#6916,0.269999999999996);
#2075=CIRCLE('',#6917,0.269999999999996);
#2076=CIRCLE('',#6919,3.68751484013273);
#2077=CIRCLE('',#6920,3.68751484013274);
#2078=CIRCLE('',#6922,0.27);
#2079=CIRCLE('',#6923,0.27);
#2080=CIRCLE('',#6925,3.68751484013274);
#2081=CIRCLE('',#6926,3.68751484013274);
#2082=CIRCLE('',#6928,0.269999999999999);
#2083=CIRCLE('',#6929,0.269999999999999);
#2084=CIRCLE('',#6931,0.269999999999999);
#2085=CIRCLE('',#6932,0.269999999999999);
#2086=CIRCLE('',#6934,0.270000000000005);
#2087=CIRCLE('',#6935,0.270000000000005);
#2088=CIRCLE('',#6937,0.269999999999999);
#2089=CIRCLE('',#6938,0.269999999999999);
#2090=CIRCLE('',#6940,0.269999999999999);
#2091=CIRCLE('',#6941,0.269999999999999);
#2092=CIRCLE('',#6943,0.269999999999999);
#2093=CIRCLE('',#6944,0.269999999999999);
#2094=CIRCLE('',#6946,0.269999999999999);
#2095=CIRCLE('',#6947,0.269999999999999);
#2096=CIRCLE('',#6949,0.269999999999999);
#2097=CIRCLE('',#6950,0.269999999999999);
#2098=CIRCLE('',#6952,0.269999999999999);
#2099=CIRCLE('',#6953,0.269999999999999);
#2100=CIRCLE('',#6955,0.270000000000003);
#2101=CIRCLE('',#6956,0.270000000000003);
#2102=CIRCLE('',#6958,14.3999999999983);
#2103=CIRCLE('',#6959,14.3999999999981);
#2104=CIRCLE('',#6961,14.399999999999);
#2105=CIRCLE('',#6962,14.4000000000003);
#2106=CIRCLE('',#6964,14.4000000000038);
#2107=CIRCLE('',#6965,14.4000000000017);
#2108=CIRCLE('',#6967,14.4000000000006);
#2109=CIRCLE('',#6968,14.4000000000006);
#2110=CIRCLE('',#6970,14.3999999999975);
#2111=CIRCLE('',#6971,14.4000000000014);
#2112=CIRCLE('',#6973,14.399999999997);
#2113=CIRCLE('',#6974,14.399999999997);
#2114=CIRCLE('',#6976,14.4000000000003);
#2115=CIRCLE('',#6977,14.3999999999984);
#2116=CIRCLE('',#6979,14.4);
#2117=CIRCLE('',#6980,14.4000000000003);
#2118=CIRCLE('',#6982,14.4000000000016);
#2119=CIRCLE('',#6983,14.4000000000016);
#2120=CIRCLE('',#6985,14.4000000000005);
#2121=CIRCLE('',#6986,14.4000000000001);
#2122=CIRCLE('',#6988,14.3999999999991);
#2123=CIRCLE('',#6989,14.3999999999994);
#2124=CIRCLE('',#6991,14.3999999999988);
#2125=CIRCLE('',#6992,14.3999999999988);
#2126=CIRCLE('',#6994,14.4000000000015);
#2127=CIRCLE('',#6995,14.4000000000014);
#2128=CIRCLE('',#6997,14.4000000000037);
#2129=CIRCLE('',#6998,14.4000000000039);
#2130=CIRCLE('',#7000,14.4000000000005);
#2131=CIRCLE('',#7001,14.4000000000006);
#2132=CIRCLE('',#7003,14.3999999999991);
#2133=CIRCLE('',#7004,14.3999999999995);
#2134=CIRCLE('',#7006,14.4000000000014);
#2135=CIRCLE('',#7007,14.4000000000014);
#2136=CIRCLE('',#7009,14.4000000000019);
#2137=CIRCLE('',#7010,14.4000000000005);
#2138=CIRCLE('',#7012,14.4000000000007);
#2139=CIRCLE('',#7013,14.4000000000011);
#2140=CIRCLE('',#7015,14.4000000000004);
#2141=CIRCLE('',#7016,14.4000000000004);
#2142=CIRCLE('',#7018,14.3999999999997);
#2143=CIRCLE('',#7019,14.3999999999997);
#2144=CIRCLE('',#7021,14.4000000000024);
#2145=CIRCLE('',#7022,14.4000000000024);
#2146=CIRCLE('',#7024,14.3999999999984);
#2147=CIRCLE('',#7025,14.3999999999984);
#2148=CIRCLE('',#7027,14.4000000000024);
#2149=CIRCLE('',#7028,14.4);
#2150=CIRCLE('',#7030,14.4000000000004);
#2151=CIRCLE('',#7031,14.3999999999987);
#2152=CIRCLE('',#7033,14.4000000000022);
#2153=CIRCLE('',#7034,14.4000000000021);
#2154=CIRCLE('',#7036,14.400000000003);
#2155=CIRCLE('',#7037,14.400000000002);
#2156=CIRCLE('',#7039,14.3999999999986);
#2157=CIRCLE('',#7040,14.3999999999991);
#2158=CIRCLE('',#7042,14.3999999999986);
#2159=CIRCLE('',#7043,14.3999999999986);
#2160=CIRCLE('',#7045,3.68751484013278);
#2161=CIRCLE('',#7046,0.269999999999998);
#2162=CIRCLE('',#7047,12.3749999999972);
#2163=CIRCLE('',#7048,0.270000000000001);
#2164=CIRCLE('',#7049,3.68751484013274);
#2165=CIRCLE('',#7050,3.68751484013271);
#2166=CIRCLE('',#7051,0.269999999999999);
#2167=CIRCLE('',#7052,12.3750000000014);
#2168=CIRCLE('',#7053,0.269999999999998);
#2169=CIRCLE('',#7054,3.68751484013275);
#2170=CIRCLE('',#7055,3.68751484013276);
#2171=CIRCLE('',#7056,0.270000000000001);
#2172=CIRCLE('',#7057,12.3750000000098);
#2173=CIRCLE('',#7058,0.270000000000001);
#2174=CIRCLE('',#7059,3.68751484013276);
#2175=CIRCLE('',#7060,3.68751484013274);
#2176=CIRCLE('',#7061,0.270000000000003);
#2177=CIRCLE('',#7062,12.3750000000051);
#2178=CIRCLE('',#7063,0.270000000000001);
#2179=CIRCLE('',#7064,3.68751484013274);
#2180=CIRCLE('',#7065,3.68751484013273);
#2181=CIRCLE('',#7066,0.269999999999998);
#2182=CIRCLE('',#7067,12.3749999999976);
#2183=CIRCLE('',#7068,0.269999999999999);
#2184=CIRCLE('',#7069,3.68751484013276);
#2185=CIRCLE('',#7070,3.68751484013274);
#2186=CIRCLE('',#7071,0.270000000000001);
#2187=CIRCLE('',#7072,12.3750000000045);
#2188=CIRCLE('',#7073,0.269999999999998);
#2189=CIRCLE('',#7074,3.68751484013275);
#2190=CIRCLE('',#7075,3.68751484013276);
#2191=CIRCLE('',#7076,0.269999999999999);
#2192=CIRCLE('',#7077,12.3749999999983);
#2193=CIRCLE('',#7078,0.270000000000001);
#2194=CIRCLE('',#7079,3.68751484013274);
#2195=CIRCLE('',#7080,3.68751484013275);
#2196=CIRCLE('',#7081,0.270000000000003);
#2197=CIRCLE('',#7082,12.3749999999972);
#2198=CIRCLE('',#7083,0.269999999999999);
#2199=CIRCLE('',#7084,3.68751484013273);
#2200=CIRCLE('',#7085,3.68751484013272);
#2201=CIRCLE('',#7086,0.270000000000003);
#2202=CIRCLE('',#7087,12.3750000000007);
#2203=CIRCLE('',#7088,0.270000000000001);
#2204=CIRCLE('',#7089,3.68751484013272);
#2205=CIRCLE('',#7090,3.68751484013275);
#2206=CIRCLE('',#7091,0.269999999999999);
#2207=CIRCLE('',#7092,12.3749999999991);
#2208=CIRCLE('',#7093,0.270000000000002);
#2209=CIRCLE('',#7094,3.68751484013276);
#2210=CIRCLE('',#7095,3.68751484013277);
#2211=CIRCLE('',#7096,0.27);
#2212=CIRCLE('',#7097,12.374999999999);
#2213=CIRCLE('',#7098,0.27);
#2214=CIRCLE('',#7099,3.68751484013274);
#2215=CIRCLE('',#7100,3.68751484013273);
#2216=CIRCLE('',#7101,0.270000000000002);
#2217=CIRCLE('',#7102,12.3749999999924);
#2218=CIRCLE('',#7103,0.270000000000002);
#2219=CIRCLE('',#7104,3.68751484013273);
#2220=CIRCLE('',#7105,12.3749999999951);
#2221=CIRCLE('',#7106,0.270000000000001);
#2222=CIRCLE('',#7107,3.68751484013273);
#2223=CIRCLE('',#7108,12.3750000000026);
#2224=CIRCLE('',#7109,0.269999999999999);
#2225=CIRCLE('',#7110,3.68751484013277);
#2226=CIRCLE('',#7111,3.68751484013274);
#2227=CIRCLE('',#7112,12.3750000000013);
#2228=CIRCLE('',#7113,0.269999999999999);
#2229=CIRCLE('',#7114,3.68751484013274);
#2230=CIRCLE('',#7115,3.68751484013272);
#2231=CIRCLE('',#7116,12.375);
#2232=CIRCLE('',#7117,0.269999999999999);
#2233=CIRCLE('',#7118,3.68751484013274);
#2234=CIRCLE('',#7119,3.68751484013274);
#2235=CIRCLE('',#7120,12.3750000000006);
#2236=CIRCLE('',#7121,0.269999999999999);
#2237=CIRCLE('',#7122,3.68751484013276);
#2238=CIRCLE('',#7123,3.68751484013275);
#2239=CIRCLE('',#7124,12.3749999999985);
#2240=CIRCLE('',#7125,0.270000000000001);
#2241=CIRCLE('',#7126,3.68751484013274);
#2242=CIRCLE('',#7127,3.68751484013273);
#2243=CIRCLE('',#7128,12.3750000000014);
#2244=CIRCLE('',#7129,0.270000000000001);
#2245=CIRCLE('',#7130,3.68751484013275);
#2246=CIRCLE('',#7131,3.68751484013273);
#2247=CIRCLE('',#7132,0.270000000000001);
#2248=CIRCLE('',#7133,12.3750000000053);
#2249=CIRCLE('',#7134,3.68751484013274);
#2250=CIRCLE('',#7135,3.68751484013275);
#2251=CIRCLE('',#7136,0.269999999999999);
#2252=CIRCLE('',#7137,12.3750000000023);
#2253=CIRCLE('',#7138,3.68751484013276);
#2254=CIRCLE('',#7139,3.68751484013273);
#2255=CIRCLE('',#7140,0.269999999999998);
#2256=CIRCLE('',#7141,12.3749999999973);
#2257=CIRCLE('',#7142,3.68751484013274);
#2258=CIRCLE('',#7143,3.68751484013276);
#2259=CIRCLE('',#7144,0.269999999999999);
#2260=CIRCLE('',#7145,12.3749999999999);
#2261=CIRCLE('',#7146,3.68751484013273);
#2262=CIRCLE('',#7147,3.68751484013276);
#2263=CIRCLE('',#7148,0.269999999999998);
#2264=CIRCLE('',#7149,12.3749999999996);
#2265=CIRCLE('',#7150,3.68751484013273);
#2266=CIRCLE('',#7151,3.68751484013272);
#2267=CIRCLE('',#7152,0.270000000000001);
#2268=CIRCLE('',#7153,12.3750000000059);
#2269=CIRCLE('',#7154,3.68751484013275);
#2270=CIRCLE('',#7155,0.269999999999999);
#2271=CIRCLE('',#7156,12.3750000000028);
#2272=CIRCLE('',#7157,14.3999999999998);
#2273=CIRCLE('',#7158,3.68751484013274);
#2274=CIRCLE('',#7159,0.269999999999999);
#2275=CIRCLE('',#7160,12.3749999999925);
#2276=CIRCLE('',#7161,0.269999999999996);
#2277=CIRCLE('',#7162,3.68751484013274);
#2278=CIRCLE('',#7163,3.68751484013274);
#2279=CIRCLE('',#7164,0.269999999999998);
#2280=CIRCLE('',#7165,12.3750000000028);
#2281=CIRCLE('',#7166,0.27);
#2282=CIRCLE('',#7167,3.68751484013274);
#2283=CIRCLE('',#7168,3.68751484013275);
#2284=CIRCLE('',#7169,0.269999999999999);
#2285=CIRCLE('',#7170,12.3750000000005);
#2286=CIRCLE('',#7171,0.269999999999999);
#2287=CIRCLE('',#7172,3.68751484013275);
#2288=CIRCLE('',#7173,3.68751484013275);
#2289=CIRCLE('',#7174,0.269999999999999);
#2290=CIRCLE('',#7175,12.3749999999995);
#2291=CIRCLE('',#7176,0.270000000000001);
#2292=CIRCLE('',#7177,3.68751484013273);
#2293=CIRCLE('',#7179,3.68751484013276);
#2294=CIRCLE('',#7180,3.68751484013275);
#2295=CIRCLE('',#7181,0.270000000000002);
#2296=CIRCLE('',#7182,12.3749999999995);
#2297=CIRCLE('',#7183,0.269999999999999);
#2298=CIRCLE('',#7184,3.68751484013274);
#2299=CIRCLE('',#7185,3.68751484013275);
#2300=CIRCLE('',#7186,0.269999999999999);
#2301=CIRCLE('',#7187,12.3750000000005);
#2302=CIRCLE('',#7188,0.269999999999999);
#2303=CIRCLE('',#7189,3.68751484013275);
#2304=CIRCLE('',#7190,3.68751484013275);
#2305=CIRCLE('',#7191,0.27);
#2306=CIRCLE('',#7192,12.3750000000028);
#2307=CIRCLE('',#7193,0.269999999999998);
#2308=CIRCLE('',#7194,3.68751484013275);
#2309=CIRCLE('',#7195,3.68751484013274);
#2310=CIRCLE('',#7196,0.269999999999996);
#2311=CIRCLE('',#7197,12.3749999999925);
#2312=CIRCLE('',#7198,0.269999999999999);
#2313=CIRCLE('',#7199,3.68751484013274);
#2314=CIRCLE('',#7200,14.3999999999958);
#2315=CIRCLE('',#7201,12.3750000000028);
#2316=CIRCLE('',#7202,0.269999999999999);
#2317=CIRCLE('',#7203,3.68751484013275);
#2318=CIRCLE('',#7204,12.3750000000059);
#2319=CIRCLE('',#7205,0.270000000000001);
#2320=CIRCLE('',#7206,3.68751484013271);
#2321=CIRCLE('',#7207,3.68751484013274);
#2322=CIRCLE('',#7208,12.3749999999996);
#2323=CIRCLE('',#7209,0.269999999999997);
#2324=CIRCLE('',#7210,3.68751484013275);
#2325=CIRCLE('',#7211,3.68751484013273);
#2326=CIRCLE('',#7212,12.3749999999999);
#2327=CIRCLE('',#7213,0.269999999999999);
#2328=CIRCLE('',#7214,3.68751484013275);
#2329=CIRCLE('',#7215,3.68751484013273);
#2330=CIRCLE('',#7216,12.3749999999973);
#2331=CIRCLE('',#7217,0.269999999999998);
#2332=CIRCLE('',#7218,3.68751484013274);
#2333=CIRCLE('',#7219,3.68751484013274);
#2334=CIRCLE('',#7220,12.3750000000023);
#2335=CIRCLE('',#7221,0.269999999999999);
#2336=CIRCLE('',#7222,3.68751484013275);
#2337=CIRCLE('',#7223,3.68751484013276);
#2338=CIRCLE('',#7224,12.3750000000053);
#2339=CIRCLE('',#7225,0.270000000000001);
#2340=CIRCLE('',#7226,3.68751484013274);
#2341=CIRCLE('',#7227,3.68751484013275);
#2342=CIRCLE('',#7228,0.270000000000001);
#2343=CIRCLE('',#7229,12.3750000000014);
#2344=CIRCLE('',#7230,3.68751484013273);
#2345=CIRCLE('',#7231,3.68751484013274);
#2346=CIRCLE('',#7232,0.270000000000001);
#2347=CIRCLE('',#7233,12.3749999999985);
#2348=CIRCLE('',#7234,3.68751484013275);
#2349=CIRCLE('',#7235,3.68751484013276);
#2350=CIRCLE('',#7236,0.269999999999999);
#2351=CIRCLE('',#7237,12.3750000000006);
#2352=CIRCLE('',#7238,3.68751484013272);
#2353=CIRCLE('',#7239,3.68751484013277);
#2354=CIRCLE('',#7240,0.269999999999999);
#2355=CIRCLE('',#7241,12.375);
#2356=CIRCLE('',#7242,3.68751484013274);
#2357=CIRCLE('',#7243,3.68751484013274);
#2358=CIRCLE('',#7244,0.269999999999999);
#2359=CIRCLE('',#7245,12.3750000000013);
#2360=CIRCLE('',#7246,3.68751484013273);
#2361=CIRCLE('',#7247,3.68751484013275);
#2362=CIRCLE('',#7248,0.269999999999999);
#2363=CIRCLE('',#7249,12.3750000000026);
#2364=CIRCLE('',#7250,3.68751484013273);
#2365=CIRCLE('',#7251,0.270000000000001);
#2366=CIRCLE('',#7252,12.3749999999951);
#2367=CIRCLE('',#7253,3.68751484013274);
#2368=CIRCLE('',#7254,0.270000000000002);
#2369=CIRCLE('',#7255,12.3749999999924);
#2370=CIRCLE('',#7256,0.270000000000002);
#2371=CIRCLE('',#7257,3.68751484013273);
#2372=CIRCLE('',#7258,3.68751484013274);
#2373=CIRCLE('',#7259,0.27);
#2374=CIRCLE('',#7260,12.374999999999);
#2375=CIRCLE('',#7261,0.27);
#2376=CIRCLE('',#7262,3.68751484013275);
#2377=CIRCLE('',#7263,3.68751484013276);
#2378=CIRCLE('',#7264,0.270000000000002);
#2379=CIRCLE('',#7265,12.3749999999991);
#2380=CIRCLE('',#7266,0.269999999999999);
#2381=CIRCLE('',#7267,3.68751484013275);
#2382=CIRCLE('',#7268,3.68751484013272);
#2383=CIRCLE('',#7269,0.270000000000001);
#2384=CIRCLE('',#7270,12.3750000000007);
#2385=CIRCLE('',#7271,0.270000000000003);
#2386=CIRCLE('',#7272,3.68751484013274);
#2387=CIRCLE('',#7273,3.68751484013273);
#2388=CIRCLE('',#7274,0.269999999999999);
#2389=CIRCLE('',#7275,12.3749999999972);
#2390=CIRCLE('',#7276,0.270000000000003);
#2391=CIRCLE('',#7277,3.68751484013275);
#2392=CIRCLE('',#7278,3.68751484013274);
#2393=CIRCLE('',#7279,0.270000000000001);
#2394=CIRCLE('',#7280,12.3749999999983);
#2395=CIRCLE('',#7281,0.269999999999999);
#2396=CIRCLE('',#7282,3.68751484013274);
#2397=CIRCLE('',#7283,3.68751484013275);
#2398=CIRCLE('',#7284,0.269999999999998);
#2399=CIRCLE('',#7285,12.3750000000045);
#2400=CIRCLE('',#7286,0.270000000000001);
#2401=CIRCLE('',#7287,3.68751484013272);
#2402=CIRCLE('',#7288,3.68751484013277);
#2403=CIRCLE('',#7289,0.269999999999999);
#2404=CIRCLE('',#7290,12.3749999999976);
#2405=CIRCLE('',#7291,0.269999999999998);
#2406=CIRCLE('',#7292,3.68751484013272);
#2407=CIRCLE('',#7293,3.68751484013274);
#2408=CIRCLE('',#7294,0.270000000000001);
#2409=CIRCLE('',#7295,12.3750000000051);
#2410=CIRCLE('',#7296,0.270000000000003);
#2411=CIRCLE('',#7297,3.68751484013273);
#2412=CIRCLE('',#7298,3.68751484013275);
#2413=CIRCLE('',#7299,0.270000000000001);
#2414=CIRCLE('',#7300,12.3750000000098);
#2415=CIRCLE('',#7301,0.270000000000001);
#2416=CIRCLE('',#7302,3.68751484013276);
#2417=CIRCLE('',#7303,3.68751484013275);
#2418=CIRCLE('',#7304,0.269999999999998);
#2419=CIRCLE('',#7305,12.3750000000014);
#2420=CIRCLE('',#7306,0.269999999999999);
#2421=CIRCLE('',#7307,3.68751484013272);
#2422=CIRCLE('',#7308,3.68751484013274);
#2423=CIRCLE('',#7309,0.270000000000001);
#2424=CIRCLE('',#7310,12.3749999999972);
#2425=CIRCLE('',#7311,0.269999999999998);
#2625=VERTEX_POINT('',#10300);
#2626=VERTEX_POINT('',#10301);
#2627=VERTEX_POINT('',#10303);
#2628=VERTEX_POINT('',#10305);
#2629=VERTEX_POINT('',#10309);
#2630=VERTEX_POINT('',#10310);
#2631=VERTEX_POINT('',#10312);
#2632=VERTEX_POINT('',#10314);
#2633=VERTEX_POINT('',#10318);
#2634=VERTEX_POINT('',#10320);
#2635=VERTEX_POINT('',#10324);
#2636=VERTEX_POINT('',#10325);
#2637=VERTEX_POINT('',#10327);
#2638=VERTEX_POINT('',#10329);
#2639=VERTEX_POINT('',#10333);
#2640=VERTEX_POINT('',#10335);
#2641=VERTEX_POINT('',#10339);
#2642=VERTEX_POINT('',#10340);
#2643=VERTEX_POINT('',#10342);
#2644=VERTEX_POINT('',#10344);
#2645=VERTEX_POINT('',#10348);
#2646=VERTEX_POINT('',#10350);
#2647=VERTEX_POINT('',#10354);
#2648=VERTEX_POINT('',#10355);
#2649=VERTEX_POINT('',#10357);
#2650=VERTEX_POINT('',#10359);
#2651=VERTEX_POINT('',#10363);
#2652=VERTEX_POINT('',#10365);
#2653=VERTEX_POINT('',#10369);
#2654=VERTEX_POINT('',#10370);
#2655=VERTEX_POINT('',#10372);
#2656=VERTEX_POINT('',#10374);
#2657=VERTEX_POINT('',#10378);
#2658=VERTEX_POINT('',#10379);
#2659=VERTEX_POINT('',#10381);
#2660=VERTEX_POINT('',#10383);
#2661=VERTEX_POINT('',#10387);
#2662=VERTEX_POINT('',#10388);
#2663=VERTEX_POINT('',#10390);
#2664=VERTEX_POINT('',#10392);
#2665=VERTEX_POINT('',#10396);
#2666=VERTEX_POINT('',#10397);
#2667=VERTEX_POINT('',#10399);
#2668=VERTEX_POINT('',#10401);
#2669=VERTEX_POINT('',#10405);
#2670=VERTEX_POINT('',#10406);
#2671=VERTEX_POINT('',#10408);
#2672=VERTEX_POINT('',#10410);
#2673=VERTEX_POINT('',#10414);
#2674=VERTEX_POINT('',#10415);
#2675=VERTEX_POINT('',#10417);
#2676=VERTEX_POINT('',#10419);
#2677=VERTEX_POINT('',#10423);
#2678=VERTEX_POINT('',#10424);
#2679=VERTEX_POINT('',#10426);
#2680=VERTEX_POINT('',#10428);
#2681=VERTEX_POINT('',#10432);
#2682=VERTEX_POINT('',#10433);
#2683=VERTEX_POINT('',#10435);
#2684=VERTEX_POINT('',#10437);
#2685=VERTEX_POINT('',#10441);
#2686=VERTEX_POINT('',#10442);
#2687=VERTEX_POINT('',#10444);
#2688=VERTEX_POINT('',#10446);
#2689=VERTEX_POINT('',#10450);
#2690=VERTEX_POINT('',#10451);
#2691=VERTEX_POINT('',#10453);
#2692=VERTEX_POINT('',#10455);
#2693=VERTEX_POINT('',#10459);
#2694=VERTEX_POINT('',#10460);
#2695=VERTEX_POINT('',#10462);
#2696=VERTEX_POINT('',#10464);
#2697=VERTEX_POINT('',#10468);
#2698=VERTEX_POINT('',#10469);
#2699=VERTEX_POINT('',#10471);
#2700=VERTEX_POINT('',#10473);
#2701=VERTEX_POINT('',#10477);
#2702=VERTEX_POINT('',#10478);
#2703=VERTEX_POINT('',#10480);
#2704=VERTEX_POINT('',#10482);
#2705=VERTEX_POINT('',#10486);
#2706=VERTEX_POINT('',#10487);
#2707=VERTEX_POINT('',#10489);
#2708=VERTEX_POINT('',#10491);
#2709=VERTEX_POINT('',#10495);
#2710=VERTEX_POINT('',#10496);
#2711=VERTEX_POINT('',#10498);
#2712=VERTEX_POINT('',#10500);
#2713=VERTEX_POINT('',#10504);
#2714=VERTEX_POINT('',#10505);
#2715=VERTEX_POINT('',#10507);
#2716=VERTEX_POINT('',#10509);
#2717=VERTEX_POINT('',#10513);
#2718=VERTEX_POINT('',#10514);
#2719=VERTEX_POINT('',#10516);
#2720=VERTEX_POINT('',#10518);
#2721=VERTEX_POINT('',#10522);
#2722=VERTEX_POINT('',#10523);
#2723=VERTEX_POINT('',#10525);
#2724=VERTEX_POINT('',#10527);
#2725=VERTEX_POINT('',#10531);
#2726=VERTEX_POINT('',#10532);
#2727=VERTEX_POINT('',#10534);
#2728=VERTEX_POINT('',#10536);
#2729=VERTEX_POINT('',#10540);
#2730=VERTEX_POINT('',#10541);
#2731=VERTEX_POINT('',#10543);
#2732=VERTEX_POINT('',#10545);
#2733=VERTEX_POINT('',#10549);
#2734=VERTEX_POINT('',#10550);
#2735=VERTEX_POINT('',#10552);
#2736=VERTEX_POINT('',#10554);
#2737=VERTEX_POINT('',#10558);
#2738=VERTEX_POINT('',#10559);
#2739=VERTEX_POINT('',#10561);
#2740=VERTEX_POINT('',#10563);
#2741=VERTEX_POINT('',#10567);
#2742=VERTEX_POINT('',#10568);
#2743=VERTEX_POINT('',#10570);
#2744=VERTEX_POINT('',#10572);
#2745=VERTEX_POINT('',#10576);
#2746=VERTEX_POINT('',#10577);
#2747=VERTEX_POINT('',#10579);
#2748=VERTEX_POINT('',#10581);
#2749=VERTEX_POINT('',#10585);
#2750=VERTEX_POINT('',#10587);
#2751=VERTEX_POINT('',#10591);
#2752=VERTEX_POINT('',#10593);
#2753=VERTEX_POINT('',#10597);
#2754=VERTEX_POINT('',#10599);
#2755=VERTEX_POINT('',#10603);
#2756=VERTEX_POINT('',#10604);
#2757=VERTEX_POINT('',#10606);
#2758=VERTEX_POINT('',#10608);
#2759=VERTEX_POINT('',#10612);
#2760=VERTEX_POINT('',#10613);
#2761=VERTEX_POINT('',#10615);
#2762=VERTEX_POINT('',#10617);
#2763=VERTEX_POINT('',#10621);
#2764=VERTEX_POINT('',#10622);
#2765=VERTEX_POINT('',#10624);
#2766=VERTEX_POINT('',#10626);
#2767=VERTEX_POINT('',#10630);
#2768=VERTEX_POINT('',#10631);
#2769=VERTEX_POINT('',#10633);
#2770=VERTEX_POINT('',#10635);
#2771=VERTEX_POINT('',#10639);
#2772=VERTEX_POINT('',#10640);
#2773=VERTEX_POINT('',#10642);
#2774=VERTEX_POINT('',#10644);
#2775=VERTEX_POINT('',#10648);
#2776=VERTEX_POINT('',#10649);
#2777=VERTEX_POINT('',#10651);
#2778=VERTEX_POINT('',#10653);
#2779=VERTEX_POINT('',#10657);
#2780=VERTEX_POINT('',#10658);
#2781=VERTEX_POINT('',#10660);
#2782=VERTEX_POINT('',#10662);
#2783=VERTEX_POINT('',#10666);
#2784=VERTEX_POINT('',#10667);
#2785=VERTEX_POINT('',#10669);
#2786=VERTEX_POINT('',#10671);
#2787=VERTEX_POINT('',#10675);
#2788=VERTEX_POINT('',#10676);
#2789=VERTEX_POINT('',#10678);
#2790=VERTEX_POINT('',#10680);
#2791=VERTEX_POINT('',#10684);
#2792=VERTEX_POINT('',#10685);
#2793=VERTEX_POINT('',#10687);
#2794=VERTEX_POINT('',#10689);
#2795=VERTEX_POINT('',#10693);
#2796=VERTEX_POINT('',#10694);
#2797=VERTEX_POINT('',#10696);
#2798=VERTEX_POINT('',#10698);
#2799=VERTEX_POINT('',#10702);
#2800=VERTEX_POINT('',#10703);
#2801=VERTEX_POINT('',#10705);
#2802=VERTEX_POINT('',#10707);
#2803=VERTEX_POINT('',#10711);
#2804=VERTEX_POINT('',#10713);
#2805=VERTEX_POINT('',#10715);
#2806=VERTEX_POINT('',#10717);
#2807=VERTEX_POINT('',#10720);
#2808=VERTEX_POINT('',#10722);
#2809=VERTEX_POINT('',#10724);
#2810=VERTEX_POINT('',#10726);
#2811=VERTEX_POINT('',#10729);
#2812=VERTEX_POINT('',#10731);
#2813=VERTEX_POINT('',#10733);
#2814=VERTEX_POINT('',#10735);
#2815=VERTEX_POINT('',#10738);
#2816=VERTEX_POINT('',#10740);
#2817=VERTEX_POINT('',#10742);
#2818=VERTEX_POINT('',#10744);
#2819=VERTEX_POINT('',#10747);
#2820=VERTEX_POINT('',#10749);
#2821=VERTEX_POINT('',#10751);
#2822=VERTEX_POINT('',#10753);
#2823=VERTEX_POINT('',#10756);
#2824=VERTEX_POINT('',#10758);
#2825=VERTEX_POINT('',#10760);
#2826=VERTEX_POINT('',#10762);
#2827=VERTEX_POINT('',#10765);
#2828=VERTEX_POINT('',#10767);
#2829=VERTEX_POINT('',#10769);
#2830=VERTEX_POINT('',#10771);
#2831=VERTEX_POINT('',#10774);
#2832=VERTEX_POINT('',#10776);
#2833=VERTEX_POINT('',#10778);
#2834=VERTEX_POINT('',#10780);
#2835=VERTEX_POINT('',#10783);
#2836=VERTEX_POINT('',#10785);
#2837=VERTEX_POINT('',#10787);
#2838=VERTEX_POINT('',#10789);
#2839=VERTEX_POINT('',#10792);
#2840=VERTEX_POINT('',#10794);
#2841=VERTEX_POINT('',#10796);
#2842=VERTEX_POINT('',#10798);
#2843=VERTEX_POINT('',#10801);
#2844=VERTEX_POINT('',#10803);
#2845=VERTEX_POINT('',#10805);
#2846=VERTEX_POINT('',#10807);
#2847=VERTEX_POINT('',#10810);
#2848=VERTEX_POINT('',#10812);
#2849=VERTEX_POINT('',#10814);
#2850=VERTEX_POINT('',#10816);
#2851=VERTEX_POINT('',#10819);
#2852=VERTEX_POINT('',#10821);
#2853=VERTEX_POINT('',#10824);
#2854=VERTEX_POINT('',#10826);
#2855=VERTEX_POINT('',#10830);
#2856=VERTEX_POINT('',#10832);
#2857=VERTEX_POINT('',#10836);
#2858=VERTEX_POINT('',#10838);
#2859=VERTEX_POINT('',#10842);
#2860=VERTEX_POINT('',#10844);
#2861=VERTEX_POINT('',#10848);
#2862=VERTEX_POINT('',#10850);
#2863=VERTEX_POINT('',#10854);
#2864=VERTEX_POINT('',#10856);
#2865=VERTEX_POINT('',#10859);
#2866=VERTEX_POINT('',#10861);
#2867=VERTEX_POINT('',#10865);
#2868=VERTEX_POINT('',#10867);
#2869=VERTEX_POINT('',#10871);
#2870=VERTEX_POINT('',#10873);
#2871=VERTEX_POINT('',#10877);
#2872=VERTEX_POINT('',#10879);
#2873=VERTEX_POINT('',#10883);
#2874=VERTEX_POINT('',#10885);
#2875=VERTEX_POINT('',#10889);
#2876=VERTEX_POINT('',#10891);
#2877=VERTEX_POINT('',#10894);
#2878=VERTEX_POINT('',#10896);
#2879=VERTEX_POINT('',#10899);
#2880=VERTEX_POINT('',#10901);
#2881=VERTEX_POINT('',#10903);
#2882=VERTEX_POINT('',#10905);
#2883=VERTEX_POINT('',#10907);
#2884=VERTEX_POINT('',#10910);
#2885=VERTEX_POINT('',#10912);
#2886=VERTEX_POINT('',#10914);
#2887=VERTEX_POINT('',#10916);
#2888=VERTEX_POINT('',#10919);
#2889=VERTEX_POINT('',#10921);
#2890=VERTEX_POINT('',#10923);
#2891=VERTEX_POINT('',#10925);
#2892=VERTEX_POINT('',#10928);
#2893=VERTEX_POINT('',#10930);
#2894=VERTEX_POINT('',#10932);
#2895=VERTEX_POINT('',#10934);
#2896=VERTEX_POINT('',#10937);
#2897=VERTEX_POINT('',#10939);
#2898=VERTEX_POINT('',#10943);
#2899=VERTEX_POINT('',#10945);
#2900=VERTEX_POINT('',#10947);
#2901=VERTEX_POINT('',#10949);
#2902=VERTEX_POINT('',#10951);
#2903=VERTEX_POINT('',#10954);
#2904=VERTEX_POINT('',#10956);
#2905=VERTEX_POINT('',#10958);
#2906=VERTEX_POINT('',#10960);
#2907=VERTEX_POINT('',#10963);
#2908=VERTEX_POINT('',#10965);
#2909=VERTEX_POINT('',#10967);
#2910=VERTEX_POINT('',#10969);
#2911=VERTEX_POINT('',#10972);
#2912=VERTEX_POINT('',#10974);
#2913=VERTEX_POINT('',#10976);
#2914=VERTEX_POINT('',#10978);
#2915=VERTEX_POINT('',#10980);
#2916=VERTEX_POINT('',#10983);
#2917=VERTEX_POINT('',#10985);
#2918=VERTEX_POINT('',#10988);
#2919=VERTEX_POINT('',#10990);
#2920=VERTEX_POINT('',#10994);
#2921=VERTEX_POINT('',#10996);
#2922=VERTEX_POINT('',#11000);
#2923=VERTEX_POINT('',#11002);
#2924=VERTEX_POINT('',#11006);
#2925=VERTEX_POINT('',#11008);
#2926=VERTEX_POINT('',#11012);
#2927=VERTEX_POINT('',#11014);
#2928=VERTEX_POINT('',#11018);
#2929=VERTEX_POINT('',#11020);
#2930=VERTEX_POINT('',#11023);
#2931=VERTEX_POINT('',#11025);
#2932=VERTEX_POINT('',#11029);
#2933=VERTEX_POINT('',#11031);
#2934=VERTEX_POINT('',#11035);
#2935=VERTEX_POINT('',#11037);
#2936=VERTEX_POINT('',#11041);
#2937=VERTEX_POINT('',#11043);
#2938=VERTEX_POINT('',#11047);
#2939=VERTEX_POINT('',#11049);
#2940=VERTEX_POINT('',#11053);
#2941=VERTEX_POINT('',#11055);
#2942=VERTEX_POINT('',#11058);
#2943=VERTEX_POINT('',#11060);
#2944=VERTEX_POINT('',#11063);
#2945=VERTEX_POINT('',#11065);
#2946=VERTEX_POINT('',#11067);
#2947=VERTEX_POINT('',#11069);
#2948=VERTEX_POINT('',#11072);
#2949=VERTEX_POINT('',#11074);
#2950=VERTEX_POINT('',#11076);
#2951=VERTEX_POINT('',#11078);
#2952=VERTEX_POINT('',#11081);
#2953=VERTEX_POINT('',#11083);
#2954=VERTEX_POINT('',#11085);
#2955=VERTEX_POINT('',#11087);
#2956=VERTEX_POINT('',#11090);
#2957=VERTEX_POINT('',#11092);
#2958=VERTEX_POINT('',#11094);
#2959=VERTEX_POINT('',#11096);
#2960=VERTEX_POINT('',#11099);
#2961=VERTEX_POINT('',#11101);
#2962=VERTEX_POINT('',#11103);
#2963=VERTEX_POINT('',#11105);
#2964=VERTEX_POINT('',#11108);
#2965=VERTEX_POINT('',#11110);
#2966=VERTEX_POINT('',#11112);
#2967=VERTEX_POINT('',#11114);
#2968=VERTEX_POINT('',#11117);
#2969=VERTEX_POINT('',#11119);
#2970=VERTEX_POINT('',#11121);
#2971=VERTEX_POINT('',#11123);
#2972=VERTEX_POINT('',#11126);
#2973=VERTEX_POINT('',#11128);
#2974=VERTEX_POINT('',#11130);
#2975=VERTEX_POINT('',#11132);
#2976=VERTEX_POINT('',#11135);
#2977=VERTEX_POINT('',#11137);
#2978=VERTEX_POINT('',#11139);
#2979=VERTEX_POINT('',#11141);
#2980=VERTEX_POINT('',#11144);
#2981=VERTEX_POINT('',#11146);
#2982=VERTEX_POINT('',#11148);
#2983=VERTEX_POINT('',#11150);
#2984=VERTEX_POINT('',#11153);
#2985=VERTEX_POINT('',#11155);
#2986=VERTEX_POINT('',#11157);
#2987=VERTEX_POINT('',#11159);
#2988=VERTEX_POINT('',#11162);
#2989=VERTEX_POINT('',#11164);
#2990=VERTEX_POINT('',#11166);
#2991=VERTEX_POINT('',#11169);
#2992=VERTEX_POINT('',#11171);
#3332=EDGE_CURVE('',#2625,#2626,#2064,.T.);
#3333=EDGE_CURVE('',#2625,#2627,#1191,.T.);
#3334=EDGE_CURVE('',#2627,#2628,#2065,.T.);
#3335=EDGE_CURVE('',#2626,#2628,#1192,.T.);
#3336=EDGE_CURVE('',#2629,#2630,#2066,.T.);
#3337=EDGE_CURVE('',#2631,#2629,#1193,.T.);
#3338=EDGE_CURVE('',#2632,#2631,#2067,.T.);
#3339=EDGE_CURVE('',#2630,#2632,#1194,.T.);
#3340=EDGE_CURVE('',#2633,#2632,#2068,.T.);
#3341=EDGE_CURVE('',#2634,#2633,#1195,.T.);
#3342=EDGE_CURVE('',#2634,#2630,#2069,.T.);
#3343=EDGE_CURVE('',#2635,#2636,#2070,.T.);
#3344=EDGE_CURVE('',#2637,#2635,#1196,.T.);
#3345=EDGE_CURVE('',#2638,#2637,#2071,.T.);
#3346=EDGE_CURVE('',#2636,#2638,#1197,.T.);
#3347=EDGE_CURVE('',#2639,#2638,#2072,.T.);
#3348=EDGE_CURVE('',#2640,#2639,#1198,.T.);
#3349=EDGE_CURVE('',#2640,#2636,#2073,.T.);
#3350=EDGE_CURVE('',#2641,#2642,#2074,.T.);
#3351=EDGE_CURVE('',#2643,#2641,#1199,.T.);
#3352=EDGE_CURVE('',#2644,#2643,#2075,.T.);
#3353=EDGE_CURVE('',#2642,#2644,#1200,.T.);
#3354=EDGE_CURVE('',#2643,#2645,#2076,.T.);
#3355=EDGE_CURVE('',#2641,#2646,#2077,.T.);
#3356=EDGE_CURVE('',#2645,#2646,#1201,.T.);
#3357=EDGE_CURVE('',#2647,#2648,#2078,.T.);
#3358=EDGE_CURVE('',#2649,#2647,#1202,.T.);
#3359=EDGE_CURVE('',#2650,#2649,#2079,.T.);
#3360=EDGE_CURVE('',#2648,#2650,#1203,.T.);
#3361=EDGE_CURVE('',#2649,#2651,#2080,.T.);
#3362=EDGE_CURVE('',#2647,#2652,#2081,.T.);
#3363=EDGE_CURVE('',#2651,#2652,#1204,.T.);
#3364=EDGE_CURVE('',#2653,#2654,#2082,.T.);
#3365=EDGE_CURVE('',#2655,#2653,#1205,.T.);
#3366=EDGE_CURVE('',#2656,#2655,#2083,.T.);
#3367=EDGE_CURVE('',#2654,#2656,#1206,.T.);
#3368=EDGE_CURVE('',#2657,#2658,#2084,.T.);
#3369=EDGE_CURVE('',#2659,#2657,#1207,.T.);
#3370=EDGE_CURVE('',#2660,#2659,#2085,.T.);
#3371=EDGE_CURVE('',#2658,#2660,#1208,.T.);
#3372=EDGE_CURVE('',#2661,#2662,#2086,.T.);
#3373=EDGE_CURVE('',#2663,#2661,#1209,.T.);
#3374=EDGE_CURVE('',#2664,#2663,#2087,.T.);
#3375=EDGE_CURVE('',#2662,#2664,#1210,.T.);
#3376=EDGE_CURVE('',#2665,#2666,#2088,.T.);
#3377=EDGE_CURVE('',#2667,#2665,#1211,.T.);
#3378=EDGE_CURVE('',#2668,#2667,#2089,.T.);
#3379=EDGE_CURVE('',#2666,#2668,#1212,.T.);
#3380=EDGE_CURVE('',#2669,#2670,#2090,.T.);
#3381=EDGE_CURVE('',#2671,#2669,#1213,.T.);
#3382=EDGE_CURVE('',#2672,#2671,#2091,.T.);
#3383=EDGE_CURVE('',#2670,#2672,#1214,.T.);
#3384=EDGE_CURVE('',#2673,#2674,#2092,.T.);
#3385=EDGE_CURVE('',#2675,#2673,#1215,.T.);
#3386=EDGE_CURVE('',#2676,#2675,#2093,.T.);
#3387=EDGE_CURVE('',#2674,#2676,#1216,.T.);
#3388=EDGE_CURVE('',#2677,#2678,#2094,.T.);
#3389=EDGE_CURVE('',#2679,#2677,#1217,.T.);
#3390=EDGE_CURVE('',#2680,#2679,#2095,.T.);
#3391=EDGE_CURVE('',#2678,#2680,#1218,.T.);
#3392=EDGE_CURVE('',#2681,#2682,#2096,.T.);
#3393=EDGE_CURVE('',#2683,#2681,#1219,.T.);
#3394=EDGE_CURVE('',#2684,#2683,#2097,.T.);
#3395=EDGE_CURVE('',#2682,#2684,#1220,.T.);
#3396=EDGE_CURVE('',#2685,#2686,#2098,.T.);
#3397=EDGE_CURVE('',#2687,#2685,#1221,.T.);
#3398=EDGE_CURVE('',#2688,#2687,#2099,.T.);
#3399=EDGE_CURVE('',#2686,#2688,#1222,.T.);
#3400=EDGE_CURVE('',#2689,#2690,#2100,.T.);
#3401=EDGE_CURVE('',#2691,#2689,#1223,.T.);
#3402=EDGE_CURVE('',#2692,#2691,#2101,.T.);
#3403=EDGE_CURVE('',#2690,#2692,#1224,.T.);
#3404=EDGE_CURVE('',#2693,#2694,#2102,.T.);
#3405=EDGE_CURVE('',#2693,#2695,#1225,.T.);
#3406=EDGE_CURVE('',#2695,#2696,#2103,.T.);
#3407=EDGE_CURVE('',#2696,#2694,#1226,.T.);
#3408=EDGE_CURVE('',#2697,#2698,#2104,.T.);
#3409=EDGE_CURVE('',#2697,#2699,#1227,.T.);
#3410=EDGE_CURVE('',#2699,#2700,#2105,.T.);
#3411=EDGE_CURVE('',#2700,#2698,#1228,.T.);
#3412=EDGE_CURVE('',#2701,#2702,#2106,.T.);
#3413=EDGE_CURVE('',#2702,#2703,#1229,.T.);
#3414=EDGE_CURVE('',#2704,#2703,#2107,.T.);
#3415=EDGE_CURVE('',#2704,#2701,#1230,.T.);
#3416=EDGE_CURVE('',#2705,#2706,#2108,.T.);
#3417=EDGE_CURVE('',#2705,#2707,#1231,.T.);
#3418=EDGE_CURVE('',#2707,#2708,#2109,.T.);
#3419=EDGE_CURVE('',#2708,#2706,#1232,.T.);
#3420=EDGE_CURVE('',#2709,#2710,#2110,.T.);
#3421=EDGE_CURVE('',#2709,#2711,#1233,.T.);
#3422=EDGE_CURVE('',#2711,#2712,#2111,.T.);
#3423=EDGE_CURVE('',#2712,#2710,#1234,.T.);
#3424=EDGE_CURVE('',#2713,#2714,#2112,.T.);
#3425=EDGE_CURVE('',#2714,#2715,#1235,.T.);
#3426=EDGE_CURVE('',#2716,#2715,#2113,.T.);
#3427=EDGE_CURVE('',#2716,#2713,#1236,.T.);
#3428=EDGE_CURVE('',#2717,#2718,#2114,.T.);
#3429=EDGE_CURVE('',#2718,#2719,#1237,.T.);
#3430=EDGE_CURVE('',#2720,#2719,#2115,.T.);
#3431=EDGE_CURVE('',#2720,#2717,#1238,.T.);
#3432=EDGE_CURVE('',#2721,#2722,#2116,.T.);
#3433=EDGE_CURVE('',#2722,#2723,#1239,.T.);
#3434=EDGE_CURVE('',#2724,#2723,#2117,.T.);
#3435=EDGE_CURVE('',#2724,#2721,#1240,.T.);
#3436=EDGE_CURVE('',#2725,#2726,#2118,.T.);
#3437=EDGE_CURVE('',#2725,#2727,#1241,.T.);
#3438=EDGE_CURVE('',#2727,#2728,#2119,.T.);
#3439=EDGE_CURVE('',#2728,#2726,#1242,.T.);
#3440=EDGE_CURVE('',#2729,#2730,#2120,.T.);
#3441=EDGE_CURVE('',#2729,#2731,#1243,.T.);
#3442=EDGE_CURVE('',#2731,#2732,#2121,.T.);
#3443=EDGE_CURVE('',#2732,#2730,#1244,.T.);
#3444=EDGE_CURVE('',#2733,#2734,#2122,.T.);
#3445=EDGE_CURVE('',#2734,#2735,#1245,.T.);
#3446=EDGE_CURVE('',#2736,#2735,#2123,.T.);
#3447=EDGE_CURVE('',#2736,#2733,#1246,.T.);
#3448=EDGE_CURVE('',#2737,#2738,#2124,.T.);
#3449=EDGE_CURVE('',#2738,#2739,#1247,.T.);
#3450=EDGE_CURVE('',#2740,#2739,#2125,.T.);
#3451=EDGE_CURVE('',#2740,#2737,#1248,.T.);
#3452=EDGE_CURVE('',#2741,#2742,#2126,.T.);
#3453=EDGE_CURVE('',#2742,#2743,#1249,.T.);
#3454=EDGE_CURVE('',#2744,#2743,#2127,.T.);
#3455=EDGE_CURVE('',#2744,#2741,#1250,.T.);
#3456=EDGE_CURVE('',#2745,#2746,#2128,.T.);
#3457=EDGE_CURVE('',#2746,#2747,#1251,.T.);
#3458=EDGE_CURVE('',#2748,#2747,#2129,.T.);
#3459=EDGE_CURVE('',#2748,#2745,#1252,.T.);
#3460=EDGE_CURVE('',#2633,#2749,#2130,.T.);
#3461=EDGE_CURVE('',#2749,#2750,#1253,.T.);
#3462=EDGE_CURVE('',#2634,#2750,#2131,.T.);
#3463=EDGE_CURVE('',#2639,#2751,#2132,.T.);
#3464=EDGE_CURVE('',#2751,#2752,#1254,.T.);
#3465=EDGE_CURVE('',#2640,#2752,#2133,.T.);
#3466=EDGE_CURVE('',#2753,#2652,#2134,.T.);
#3467=EDGE_CURVE('',#2753,#2754,#1255,.T.);
#3468=EDGE_CURVE('',#2754,#2651,#2135,.T.);
#3469=EDGE_CURVE('',#2755,#2756,#2136,.T.);
#3470=EDGE_CURVE('',#2755,#2757,#1256,.T.);
#3471=EDGE_CURVE('',#2757,#2758,#2137,.T.);
#3472=EDGE_CURVE('',#2758,#2756,#1257,.T.);
#3473=EDGE_CURVE('',#2759,#2760,#2138,.T.);
#3474=EDGE_CURVE('',#2759,#2761,#1258,.T.);
#3475=EDGE_CURVE('',#2761,#2762,#2139,.T.);
#3476=EDGE_CURVE('',#2762,#2760,#1259,.T.);
#3477=EDGE_CURVE('',#2763,#2764,#2140,.T.);
#3478=EDGE_CURVE('',#2764,#2765,#1260,.T.);
#3479=EDGE_CURVE('',#2766,#2765,#2141,.T.);
#3480=EDGE_CURVE('',#2766,#2763,#1261,.T.);
#3481=EDGE_CURVE('',#2767,#2768,#2142,.T.);
#3482=EDGE_CURVE('',#2767,#2769,#1262,.T.);
#3483=EDGE_CURVE('',#2769,#2770,#2143,.T.);
#3484=EDGE_CURVE('',#2770,#2768,#1263,.T.);
#3485=EDGE_CURVE('',#2771,#2772,#2144,.T.);
#3486=EDGE_CURVE('',#2771,#2773,#1264,.T.);
#3487=EDGE_CURVE('',#2773,#2774,#2145,.T.);
#3488=EDGE_CURVE('',#2774,#2772,#1265,.T.);
#3489=EDGE_CURVE('',#2775,#2776,#2146,.T.);
#3490=EDGE_CURVE('',#2775,#2777,#1266,.T.);
#3491=EDGE_CURVE('',#2777,#2778,#2147,.T.);
#3492=EDGE_CURVE('',#2778,#2776,#1267,.T.);
#3493=EDGE_CURVE('',#2779,#2780,#2148,.T.);
#3494=EDGE_CURVE('',#2779,#2781,#1268,.T.);
#3495=EDGE_CURVE('',#2781,#2782,#2149,.T.);
#3496=EDGE_CURVE('',#2782,#2780,#1269,.T.);
#3497=EDGE_CURVE('',#2783,#2784,#2150,.T.);
#3498=EDGE_CURVE('',#2783,#2785,#1270,.T.);
#3499=EDGE_CURVE('',#2785,#2786,#2151,.T.);
#3500=EDGE_CURVE('',#2786,#2784,#1271,.T.);
#3501=EDGE_CURVE('',#2787,#2788,#2152,.T.);
#3502=EDGE_CURVE('',#2788,#2789,#1272,.T.);
#3503=EDGE_CURVE('',#2790,#2789,#2153,.T.);
#3504=EDGE_CURVE('',#2790,#2787,#1273,.T.);
#3505=EDGE_CURVE('',#2791,#2792,#2154,.T.);
#3506=EDGE_CURVE('',#2792,#2793,#1274,.T.);
#3507=EDGE_CURVE('',#2794,#2793,#2155,.T.);
#3508=EDGE_CURVE('',#2794,#2791,#1275,.T.);
#3509=EDGE_CURVE('',#2795,#2796,#2156,.T.);
#3510=EDGE_CURVE('',#2796,#2797,#1276,.T.);
#3511=EDGE_CURVE('',#2798,#2797,#2157,.T.);
#3512=EDGE_CURVE('',#2798,#2795,#1277,.T.);
#3513=EDGE_CURVE('',#2799,#2800,#2158,.T.);
#3514=EDGE_CURVE('',#2799,#2801,#1278,.T.);
#3515=EDGE_CURVE('',#2801,#2802,#2159,.T.);
#3516=EDGE_CURVE('',#2802,#2800,#1279,.T.);
#3517=EDGE_CURVE('',#2699,#2803,#2160,.T.);
#3518=EDGE_CURVE('',#2803,#2804,#2161,.T.);
#3519=EDGE_CURVE('',#2804,#2805,#2162,.T.);
#3520=EDGE_CURVE('',#2805,#2806,#2163,.T.);
#3521=EDGE_CURVE('',#2806,#2702,#2164,.T.);
#3522=EDGE_CURVE('',#2701,#2807,#2165,.T.);
#3523=EDGE_CURVE('',#2807,#2808,#2166,.T.);
#3524=EDGE_CURVE('',#2808,#2809,#2167,.T.);
#3525=EDGE_CURVE('',#2809,#2810,#2168,.T.);
#3526=EDGE_CURVE('',#2810,#2714,#2169,.T.);
#3527=EDGE_CURVE('',#2713,#2811,#2170,.T.);
#3528=EDGE_CURVE('',#2811,#2812,#2171,.T.);
#3529=EDGE_CURVE('',#2812,#2813,#2172,.T.);
#3530=EDGE_CURVE('',#2813,#2814,#2173,.T.);
#3531=EDGE_CURVE('',#2814,#2718,#2174,.T.);
#3532=EDGE_CURVE('',#2717,#2815,#2175,.T.);
#3533=EDGE_CURVE('',#2815,#2816,#2176,.T.);
#3534=EDGE_CURVE('',#2816,#2817,#2177,.T.);
#3535=EDGE_CURVE('',#2817,#2818,#2178,.T.);
#3536=EDGE_CURVE('',#2818,#2696,#2179,.T.);
#3537=EDGE_CURVE('',#2695,#2819,#2180,.T.);
#3538=EDGE_CURVE('',#2819,#2820,#2181,.T.);
#3539=EDGE_CURVE('',#2820,#2821,#2182,.T.);
#3540=EDGE_CURVE('',#2821,#2822,#2183,.T.);
#3541=EDGE_CURVE('',#2822,#2722,#2184,.T.);
#3542=EDGE_CURVE('',#2721,#2823,#2185,.T.);
#3543=EDGE_CURVE('',#2823,#2824,#2186,.T.);
#3544=EDGE_CURVE('',#2824,#2825,#2187,.T.);
#3545=EDGE_CURVE('',#2825,#2826,#2188,.T.);
#3546=EDGE_CURVE('',#2826,#2734,#2189,.T.);
#3547=EDGE_CURVE('',#2733,#2827,#2190,.T.);
#3548=EDGE_CURVE('',#2827,#2828,#2191,.T.);
#3549=EDGE_CURVE('',#2828,#2829,#2192,.T.);
#3550=EDGE_CURVE('',#2829,#2830,#2193,.T.);
#3551=EDGE_CURVE('',#2830,#2738,#2194,.T.);
#3552=EDGE_CURVE('',#2737,#2831,#2195,.T.);
#3553=EDGE_CURVE('',#2831,#2832,#2196,.T.);
#3554=EDGE_CURVE('',#2832,#2833,#2197,.T.);
#3555=EDGE_CURVE('',#2833,#2834,#2198,.T.);
#3556=EDGE_CURVE('',#2834,#2732,#2199,.T.);
#3557=EDGE_CURVE('',#2731,#2835,#2200,.T.);
#3558=EDGE_CURVE('',#2835,#2836,#2201,.T.);
#3559=EDGE_CURVE('',#2836,#2837,#2202,.T.);
#3560=EDGE_CURVE('',#2837,#2838,#2203,.T.);
#3561=EDGE_CURVE('',#2838,#2728,#2204,.T.);
#3562=EDGE_CURVE('',#2727,#2839,#2205,.T.);
#3563=EDGE_CURVE('',#2839,#2840,#2206,.T.);
#3564=EDGE_CURVE('',#2840,#2841,#2207,.T.);
#3565=EDGE_CURVE('',#2841,#2842,#2208,.T.);
#3566=EDGE_CURVE('',#2842,#2742,#2209,.T.);
#3567=EDGE_CURVE('',#2741,#2843,#2210,.T.);
#3568=EDGE_CURVE('',#2843,#2844,#2211,.T.);
#3569=EDGE_CURVE('',#2844,#2845,#2212,.T.);
#3570=EDGE_CURVE('',#2845,#2846,#2213,.T.);
#3571=EDGE_CURVE('',#2846,#2746,#2214,.T.);
#3572=EDGE_CURVE('',#2745,#2847,#2215,.T.);
#3573=EDGE_CURVE('',#2847,#2848,#2216,.T.);
#3574=EDGE_CURVE('',#2848,#2849,#2217,.T.);
#3575=EDGE_CURVE('',#2849,#2850,#2218,.T.);
#3576=EDGE_CURVE('',#2850,#2749,#2219,.T.);
#3577=EDGE_CURVE('',#2631,#2851,#2220,.T.);
#3578=EDGE_CURVE('',#2851,#2852,#2221,.T.);
#3579=EDGE_CURVE('',#2852,#2751,#2222,.T.);
#3580=EDGE_CURVE('',#2637,#2853,#2223,.T.);
#3581=EDGE_CURVE('',#2853,#2854,#2224,.T.);
#3582=EDGE_CURVE('',#2854,#2788,#2225,.T.);
#3583=EDGE_CURVE('',#2787,#2684,#2226,.T.);
#3584=EDGE_CURVE('',#2683,#2855,#2227,.T.);
#3585=EDGE_CURVE('',#2855,#2856,#2228,.T.);
#3586=EDGE_CURVE('',#2856,#2786,#2229,.T.);
#3587=EDGE_CURVE('',#2785,#2680,#2230,.T.);
#3588=EDGE_CURVE('',#2679,#2857,#2231,.T.);
#3589=EDGE_CURVE('',#2857,#2858,#2232,.T.);
#3590=EDGE_CURVE('',#2858,#2792,#2233,.T.);
#3591=EDGE_CURVE('',#2791,#2688,#2234,.T.);
#3592=EDGE_CURVE('',#2687,#2859,#2235,.T.);
#3593=EDGE_CURVE('',#2859,#2860,#2236,.T.);
#3594=EDGE_CURVE('',#2860,#2796,#2237,.T.);
#3595=EDGE_CURVE('',#2795,#2692,#2238,.T.);
#3596=EDGE_CURVE('',#2691,#2861,#2239,.T.);
#3597=EDGE_CURVE('',#2861,#2862,#2240,.T.);
#3598=EDGE_CURVE('',#2862,#2782,#2241,.T.);
#3599=EDGE_CURVE('',#2781,#2676,#2242,.T.);
#3600=EDGE_CURVE('',#2675,#2863,#2243,.T.);
#3601=EDGE_CURVE('',#2863,#2864,#2244,.T.);
#3602=EDGE_CURVE('',#2864,#2778,#2245,.T.);
#3603=EDGE_CURVE('',#2777,#2865,#2246,.T.);
#3604=EDGE_CURVE('',#2865,#2866,#2247,.T.);
#3605=EDGE_CURVE('',#2866,#2672,#2248,.T.);
#3606=EDGE_CURVE('',#2671,#2774,#2249,.T.);
#3607=EDGE_CURVE('',#2773,#2867,#2250,.T.);
#3608=EDGE_CURVE('',#2867,#2868,#2251,.T.);
#3609=EDGE_CURVE('',#2868,#2668,#2252,.T.);
#3610=EDGE_CURVE('',#2667,#2770,#2253,.T.);
#3611=EDGE_CURVE('',#2769,#2869,#2254,.T.);
#3612=EDGE_CURVE('',#2869,#2870,#2255,.T.);
#3613=EDGE_CURVE('',#2870,#2664,#2256,.T.);
#3614=EDGE_CURVE('',#2663,#2762,#2257,.T.);
#3615=EDGE_CURVE('',#2761,#2871,#2258,.T.);
#3616=EDGE_CURVE('',#2871,#2872,#2259,.T.);
#3617=EDGE_CURVE('',#2872,#2656,#2260,.T.);
#3618=EDGE_CURVE('',#2655,#2764,#2261,.T.);
#3619=EDGE_CURVE('',#2763,#2873,#2262,.T.);
#3620=EDGE_CURVE('',#2873,#2874,#2263,.T.);
#3621=EDGE_CURVE('',#2874,#2660,#2264,.T.);
#3622=EDGE_CURVE('',#2659,#2758,#2265,.T.);
#3623=EDGE_CURVE('',#2757,#2875,#2266,.T.);
#3624=EDGE_CURVE('',#2875,#2876,#2267,.T.);
#3625=EDGE_CURVE('',#2876,#2650,#2268,.T.);
#3626=EDGE_CURVE('',#2754,#2877,#2269,.T.);
#3627=EDGE_CURVE('',#2877,#2878,#2270,.T.);
#3628=EDGE_CURVE('',#2878,#2644,#2271,.T.);
#3629=EDGE_CURVE('',#2879,#2645,#2272,.T.);
#3630=EDGE_CURVE('',#2879,#2880,#2273,.T.);
#3631=EDGE_CURVE('',#2880,#2881,#2274,.T.);
#3632=EDGE_CURVE('',#2881,#2882,#2275,.T.);
#3633=EDGE_CURVE('',#2882,#2883,#2276,.T.);
#3634=EDGE_CURVE('',#2883,#2802,#2277,.T.);
#3635=EDGE_CURVE('',#2801,#2884,#2278,.T.);
#3636=EDGE_CURVE('',#2884,#2885,#2279,.T.);
#3637=EDGE_CURVE('',#2885,#2886,#2280,.T.);
#3638=EDGE_CURVE('',#2886,#2887,#2281,.T.);
#3639=EDGE_CURVE('',#2887,#2712,#2282,.T.);
#3640=EDGE_CURVE('',#2711,#2888,#2283,.T.);
#3641=EDGE_CURVE('',#2888,#2889,#2284,.T.);
#3642=EDGE_CURVE('',#2889,#2890,#2285,.T.);
#3643=EDGE_CURVE('',#2890,#2891,#2286,.T.);
#3644=EDGE_CURVE('',#2891,#2708,#2287,.T.);
#3645=EDGE_CURVE('',#2707,#2892,#2288,.T.);
#3646=EDGE_CURVE('',#2892,#2893,#2289,.T.);
#3647=EDGE_CURVE('',#2893,#2894,#2290,.T.);
#3648=EDGE_CURVE('',#2894,#2895,#2291,.T.);
#3649=EDGE_CURVE('',#2895,#2700,#2292,.T.);
#3650=EDGE_CURVE('',#2896,#2625,#1280,.T.);
#3651=EDGE_CURVE('',#2626,#2897,#1281,.T.);
#3652=EDGE_CURVE('',#2897,#2896,#1282,.T.);
#3653=EDGE_CURVE('',#2697,#2898,#2293,.T.);
#3654=EDGE_CURVE('',#2899,#2698,#2294,.T.);
#3655=EDGE_CURVE('',#2899,#2900,#2295,.T.);
#3656=EDGE_CURVE('',#2901,#2900,#2296,.T.);
#3657=EDGE_CURVE('',#2901,#2902,#2297,.T.);
#3658=EDGE_CURVE('',#2705,#2902,#2298,.T.);
#3659=EDGE_CURVE('',#2903,#2706,#2299,.T.);
#3660=EDGE_CURVE('',#2903,#2904,#2300,.T.);
#3661=EDGE_CURVE('',#2905,#2904,#2301,.T.);
#3662=EDGE_CURVE('',#2905,#2906,#2302,.T.);
#3663=EDGE_CURVE('',#2709,#2906,#2303,.T.);
#3664=EDGE_CURVE('',#2907,#2710,#2304,.T.);
#3665=EDGE_CURVE('',#2907,#2908,#2305,.T.);
#3666=EDGE_CURVE('',#2909,#2908,#2306,.T.);
#3667=EDGE_CURVE('',#2909,#2910,#2307,.T.);
#3668=EDGE_CURVE('',#2799,#2910,#2308,.T.);
#3669=EDGE_CURVE('',#2911,#2800,#2309,.T.);
#3670=EDGE_CURVE('',#2911,#2912,#2310,.T.);
#3671=EDGE_CURVE('',#2913,#2912,#2311,.T.);
#3672=EDGE_CURVE('',#2913,#2914,#2312,.T.);
#3673=EDGE_CURVE('',#2915,#2914,#2313,.T.);
#3674=EDGE_CURVE('',#2915,#2646,#2314,.T.);
#3675=EDGE_CURVE('',#2916,#2642,#2315,.T.);
#3676=EDGE_CURVE('',#2916,#2917,#2316,.T.);
#3677=EDGE_CURVE('',#2753,#2917,#2317,.T.);
#3678=EDGE_CURVE('',#2918,#2648,#2318,.T.);
#3679=EDGE_CURVE('',#2918,#2919,#2319,.T.);
#3680=EDGE_CURVE('',#2755,#2919,#2320,.T.);
#3681=EDGE_CURVE('',#2657,#2756,#2321,.T.);
#3682=EDGE_CURVE('',#2920,#2658,#2322,.T.);
#3683=EDGE_CURVE('',#2920,#2921,#2323,.T.);
#3684=EDGE_CURVE('',#2766,#2921,#2324,.T.);
#3685=EDGE_CURVE('',#2653,#2765,#2325,.T.);
#3686=EDGE_CURVE('',#2922,#2654,#2326,.T.);
#3687=EDGE_CURVE('',#2922,#2923,#2327,.T.);
#3688=EDGE_CURVE('',#2759,#2923,#2328,.T.);
#3689=EDGE_CURVE('',#2661,#2760,#2329,.T.);
#3690=EDGE_CURVE('',#2924,#2662,#2330,.T.);
#3691=EDGE_CURVE('',#2924,#2925,#2331,.T.);
#3692=EDGE_CURVE('',#2767,#2925,#2332,.T.);
#3693=EDGE_CURVE('',#2665,#2768,#2333,.T.);
#3694=EDGE_CURVE('',#2926,#2666,#2334,.T.);
#3695=EDGE_CURVE('',#2926,#2927,#2335,.T.);
#3696=EDGE_CURVE('',#2771,#2927,#2336,.T.);
#3697=EDGE_CURVE('',#2669,#2772,#2337,.T.);
#3698=EDGE_CURVE('',#2928,#2670,#2338,.T.);
#3699=EDGE_CURVE('',#2928,#2929,#2339,.T.);
#3700=EDGE_CURVE('',#2775,#2929,#2340,.T.);
#3701=EDGE_CURVE('',#2930,#2776,#2341,.T.);
#3702=EDGE_CURVE('',#2930,#2931,#2342,.T.);
#3703=EDGE_CURVE('',#2673,#2931,#2343,.T.);
#3704=EDGE_CURVE('',#2779,#2674,#2344,.T.);
#3705=EDGE_CURVE('',#2932,#2780,#2345,.T.);
#3706=EDGE_CURVE('',#2932,#2933,#2346,.T.);
#3707=EDGE_CURVE('',#2689,#2933,#2347,.T.);
#3708=EDGE_CURVE('',#2798,#2690,#2348,.T.);
#3709=EDGE_CURVE('',#2934,#2797,#2349,.T.);
#3710=EDGE_CURVE('',#2934,#2935,#2350,.T.);
#3711=EDGE_CURVE('',#2685,#2935,#2351,.T.);
#3712=EDGE_CURVE('',#2794,#2686,#2352,.T.);
#3713=EDGE_CURVE('',#2936,#2793,#2353,.T.);
#3714=EDGE_CURVE('',#2936,#2937,#2354,.T.);
#3715=EDGE_CURVE('',#2677,#2937,#2355,.T.);
#3716=EDGE_CURVE('',#2783,#2678,#2356,.T.);
#3717=EDGE_CURVE('',#2938,#2784,#2357,.T.);
#3718=EDGE_CURVE('',#2938,#2939,#2358,.T.);
#3719=EDGE_CURVE('',#2681,#2939,#2359,.T.);
#3720=EDGE_CURVE('',#2790,#2682,#2360,.T.);
#3721=EDGE_CURVE('',#2940,#2789,#2361,.T.);
#3722=EDGE_CURVE('',#2940,#2941,#2362,.T.);
#3723=EDGE_CURVE('',#2635,#2941,#2363,.T.);
#3724=EDGE_CURVE('',#2942,#2752,#2364,.T.);
#3725=EDGE_CURVE('',#2942,#2943,#2365,.T.);
#3726=EDGE_CURVE('',#2629,#2943,#2366,.T.);
#3727=EDGE_CURVE('',#2944,#2750,#2367,.T.);
#3728=EDGE_CURVE('',#2944,#2945,#2368,.T.);
#3729=EDGE_CURVE('',#2946,#2945,#2369,.T.);
#3730=EDGE_CURVE('',#2946,#2947,#2370,.T.);
#3731=EDGE_CURVE('',#2748,#2947,#2371,.T.);
#3732=EDGE_CURVE('',#2948,#2747,#2372,.T.);
#3733=EDGE_CURVE('',#2948,#2949,#2373,.T.);
#3734=EDGE_CURVE('',#2950,#2949,#2374,.T.);
#3735=EDGE_CURVE('',#2950,#2951,#2375,.T.);
#3736=EDGE_CURVE('',#2744,#2951,#2376,.T.);
#3737=EDGE_CURVE('',#2952,#2743,#2377,.T.);
#3738=EDGE_CURVE('',#2952,#2953,#2378,.T.);
#3739=EDGE_CURVE('',#2954,#2953,#2379,.T.);
#3740=EDGE_CURVE('',#2954,#2955,#2380,.T.);
#3741=EDGE_CURVE('',#2725,#2955,#2381,.T.);
#3742=EDGE_CURVE('',#2956,#2726,#2382,.T.);
#3743=EDGE_CURVE('',#2956,#2957,#2383,.T.);
#3744=EDGE_CURVE('',#2958,#2957,#2384,.T.);
#3745=EDGE_CURVE('',#2958,#2959,#2385,.T.);
#3746=EDGE_CURVE('',#2729,#2959,#2386,.T.);
#3747=EDGE_CURVE('',#2960,#2730,#2387,.T.);
#3748=EDGE_CURVE('',#2960,#2961,#2388,.T.);
#3749=EDGE_CURVE('',#2962,#2961,#2389,.T.);
#3750=EDGE_CURVE('',#2962,#2963,#2390,.T.);
#3751=EDGE_CURVE('',#2740,#2963,#2391,.T.);
#3752=EDGE_CURVE('',#2964,#2739,#2392,.T.);
#3753=EDGE_CURVE('',#2964,#2965,#2393,.T.);
#3754=EDGE_CURVE('',#2966,#2965,#2394,.T.);
#3755=EDGE_CURVE('',#2966,#2967,#2395,.T.);
#3756=EDGE_CURVE('',#2736,#2967,#2396,.T.);
#3757=EDGE_CURVE('',#2968,#2735,#2397,.T.);
#3758=EDGE_CURVE('',#2968,#2969,#2398,.T.);
#3759=EDGE_CURVE('',#2970,#2969,#2399,.T.);
#3760=EDGE_CURVE('',#2970,#2971,#2400,.T.);
#3761=EDGE_CURVE('',#2724,#2971,#2401,.T.);
#3762=EDGE_CURVE('',#2972,#2723,#2402,.T.);
#3763=EDGE_CURVE('',#2972,#2973,#2403,.T.);
#3764=EDGE_CURVE('',#2974,#2973,#2404,.T.);
#3765=EDGE_CURVE('',#2974,#2975,#2405,.T.);
#3766=EDGE_CURVE('',#2693,#2975,#2406,.T.);
#3767=EDGE_CURVE('',#2976,#2694,#2407,.T.);
#3768=EDGE_CURVE('',#2976,#2977,#2408,.T.);
#3769=EDGE_CURVE('',#2978,#2977,#2409,.T.);
#3770=EDGE_CURVE('',#2978,#2979,#2410,.T.);
#3771=EDGE_CURVE('',#2720,#2979,#2411,.T.);
#3772=EDGE_CURVE('',#2980,#2719,#2412,.T.);
#3773=EDGE_CURVE('',#2980,#2981,#2413,.T.);
#3774=EDGE_CURVE('',#2982,#2981,#2414,.T.);
#3775=EDGE_CURVE('',#2982,#2983,#2415,.T.);
#3776=EDGE_CURVE('',#2716,#2983,#2416,.T.);
#3777=EDGE_CURVE('',#2984,#2715,#2417,.T.);
#3778=EDGE_CURVE('',#2984,#2985,#2418,.T.);
#3779=EDGE_CURVE('',#2986,#2985,#2419,.T.);
#3780=EDGE_CURVE('',#2986,#2987,#2420,.T.);
#3781=EDGE_CURVE('',#2704,#2987,#2421,.T.);
#3782=EDGE_CURVE('',#2988,#2703,#2422,.T.);
#3783=EDGE_CURVE('',#2988,#2989,#2423,.T.);
#3784=EDGE_CURVE('',#2990,#2989,#2424,.T.);
#3785=EDGE_CURVE('',#2990,#2898,#2425,.T.);
#3786=EDGE_CURVE('',#2991,#2627,#1283,.T.);
#3787=EDGE_CURVE('',#2992,#2991,#1284,.T.);
#3788=EDGE_CURVE('',#2628,#2992,#1285,.T.);
#3789=EDGE_CURVE('',#2915,#2879,#1286,.T.);
#3790=EDGE_CURVE('',#2883,#2911,#1287,.T.);
#3791=EDGE_CURVE('',#2914,#2880,#1288,.T.);
#3792=EDGE_CURVE('',#2912,#2882,#1289,.T.);
#3793=EDGE_CURVE('',#2881,#2913,#1290,.T.);
#3794=EDGE_CURVE('',#2910,#2884,#1291,.T.);
#3795=EDGE_CURVE('',#2887,#2907,#1292,.T.);
#3796=EDGE_CURVE('',#2908,#2886,#1293,.T.);
#3797=EDGE_CURVE('',#2885,#2909,#1294,.T.);
#3798=EDGE_CURVE('',#2862,#2932,#1295,.T.);
#3799=EDGE_CURVE('',#2933,#2861,#1296,.T.);
#3800=EDGE_CURVE('',#2860,#2934,#1297,.T.);
#3801=EDGE_CURVE('',#2935,#2859,#1298,.T.);
#3802=EDGE_CURVE('',#2856,#2938,#1299,.T.);
#3803=EDGE_CURVE('',#2939,#2855,#1300,.T.);
#3804=EDGE_CURVE('',#2858,#2936,#1301,.T.);
#3805=EDGE_CURVE('',#2937,#2857,#1302,.T.);
#3806=EDGE_CURVE('',#2864,#2930,#1303,.T.);
#3807=EDGE_CURVE('',#2931,#2863,#1304,.T.);
#3808=EDGE_CURVE('',#2929,#2865,#1305,.T.);
#3809=EDGE_CURVE('',#2866,#2928,#1306,.T.);
#3810=EDGE_CURVE('',#2927,#2867,#1307,.T.);
#3811=EDGE_CURVE('',#2868,#2926,#1308,.T.);
#3812=EDGE_CURVE('',#2925,#2869,#1309,.T.);
#3813=EDGE_CURVE('',#2870,#2924,#1310,.T.);
#3814=EDGE_CURVE('',#2921,#2873,#1311,.T.);
#3815=EDGE_CURVE('',#2874,#2920,#1312,.T.);
#3816=EDGE_CURVE('',#2923,#2871,#1313,.T.);
#3817=EDGE_CURVE('',#2872,#2922,#1314,.T.);
#3818=EDGE_CURVE('',#2919,#2875,#1315,.T.);
#3819=EDGE_CURVE('',#2876,#2918,#1316,.T.);
#3820=EDGE_CURVE('',#2917,#2877,#1317,.T.);
#3821=EDGE_CURVE('',#2878,#2916,#1318,.T.);
#3822=EDGE_CURVE('',#2854,#2940,#1319,.T.);
#3823=EDGE_CURVE('',#2941,#2853,#1320,.T.);
#3824=EDGE_CURVE('',#2852,#2942,#1321,.T.);
#3825=EDGE_CURVE('',#2943,#2851,#1322,.T.);
#3826=EDGE_CURVE('',#2947,#2847,#1323,.T.);
#3827=EDGE_CURVE('',#2850,#2944,#1324,.T.);
#3828=EDGE_CURVE('',#2945,#2849,#1325,.T.);
#3829=EDGE_CURVE('',#2848,#2946,#1326,.T.);
#3830=EDGE_CURVE('',#2951,#2843,#1327,.T.);
#3831=EDGE_CURVE('',#2846,#2948,#1328,.T.);
#3832=EDGE_CURVE('',#2949,#2845,#1329,.T.);
#3833=EDGE_CURVE('',#2844,#2950,#1330,.T.);
#3834=EDGE_CURVE('',#2963,#2831,#1331,.T.);
#3835=EDGE_CURVE('',#2834,#2960,#1332,.T.);
#3836=EDGE_CURVE('',#2961,#2833,#1333,.T.);
#3837=EDGE_CURVE('',#2832,#2962,#1334,.T.);
#3838=EDGE_CURVE('',#2967,#2827,#1335,.T.);
#3839=EDGE_CURVE('',#2830,#2964,#1336,.T.);
#3840=EDGE_CURVE('',#2965,#2829,#1337,.T.);
#3841=EDGE_CURVE('',#2828,#2966,#1338,.T.);
#3842=EDGE_CURVE('',#2959,#2835,#1339,.T.);
#3843=EDGE_CURVE('',#2838,#2956,#1340,.T.);
#3844=EDGE_CURVE('',#2957,#2837,#1341,.T.);
#3845=EDGE_CURVE('',#2836,#2958,#1342,.T.);
#3846=EDGE_CURVE('',#2955,#2839,#1343,.T.);
#3847=EDGE_CURVE('',#2842,#2952,#1344,.T.);
#3848=EDGE_CURVE('',#2953,#2841,#1345,.T.);
#3849=EDGE_CURVE('',#2840,#2954,#1346,.T.);
#3850=EDGE_CURVE('',#2971,#2823,#1347,.T.);
#3851=EDGE_CURVE('',#2826,#2968,#1348,.T.);
#3852=EDGE_CURVE('',#2969,#2825,#1349,.T.);
#3853=EDGE_CURVE('',#2824,#2970,#1350,.T.);
#3854=EDGE_CURVE('',#2975,#2819,#1351,.T.);
#3855=EDGE_CURVE('',#2822,#2972,#1352,.T.);
#3856=EDGE_CURVE('',#2973,#2821,#1353,.T.);
#3857=EDGE_CURVE('',#2820,#2974,#1354,.T.);
#3858=EDGE_CURVE('',#2979,#2815,#1355,.T.);
#3859=EDGE_CURVE('',#2818,#2976,#1356,.T.);
#3860=EDGE_CURVE('',#2977,#2817,#1357,.T.);
#3861=EDGE_CURVE('',#2816,#2978,#1358,.T.);
#3862=EDGE_CURVE('',#2983,#2811,#1359,.T.);
#3863=EDGE_CURVE('',#2814,#2980,#1360,.T.);
#3864=EDGE_CURVE('',#2981,#2813,#1361,.T.);
#3865=EDGE_CURVE('',#2812,#2982,#1362,.T.);
#3866=EDGE_CURVE('',#2906,#2888,#1363,.T.);
#3867=EDGE_CURVE('',#2891,#2903,#1364,.T.);
#3868=EDGE_CURVE('',#2904,#2890,#1365,.T.);
#3869=EDGE_CURVE('',#2889,#2905,#1366,.T.);
#3870=EDGE_CURVE('',#2902,#2892,#1367,.T.);
#3871=EDGE_CURVE('',#2895,#2899,#1368,.T.);
#3872=EDGE_CURVE('',#2900,#2894,#1369,.T.);
#3873=EDGE_CURVE('',#2893,#2901,#1370,.T.);
#3874=EDGE_CURVE('',#2987,#2807,#1371,.T.);
#3875=EDGE_CURVE('',#2810,#2984,#1372,.T.);
#3876=EDGE_CURVE('',#2985,#2809,#1373,.T.);
#3877=EDGE_CURVE('',#2808,#2986,#1374,.T.);
#3878=EDGE_CURVE('',#2898,#2803,#1375,.T.);
#3879=EDGE_CURVE('',#2806,#2988,#1376,.T.);
#3880=EDGE_CURVE('',#2989,#2805,#1377,.T.);
#3881=EDGE_CURVE('',#2804,#2990,#1378,.T.);
#3882=EDGE_CURVE('',#2896,#2991,#1379,.T.);
#3883=EDGE_CURVE('',#2897,#2992,#1380,.T.);
#4486=ORIENTED_EDGE('',*,*,#3332,.F.);
#4487=ORIENTED_EDGE('',*,*,#3333,.T.);
#4488=ORIENTED_EDGE('',*,*,#3334,.T.);
#4489=ORIENTED_EDGE('',*,*,#3335,.F.);
#4490=ORIENTED_EDGE('',*,*,#3336,.F.);
#4491=ORIENTED_EDGE('',*,*,#3337,.F.);
#4492=ORIENTED_EDGE('',*,*,#3338,.F.);
#4493=ORIENTED_EDGE('',*,*,#3339,.F.);
#4494=ORIENTED_EDGE('',*,*,#3340,.F.);
#4495=ORIENTED_EDGE('',*,*,#3341,.F.);
#4496=ORIENTED_EDGE('',*,*,#3342,.T.);
#4497=ORIENTED_EDGE('',*,*,#3339,.T.);
#4498=ORIENTED_EDGE('',*,*,#3343,.F.);
#4499=ORIENTED_EDGE('',*,*,#3344,.F.);
#4500=ORIENTED_EDGE('',*,*,#3345,.F.);
#4501=ORIENTED_EDGE('',*,*,#3346,.F.);
#4502=ORIENTED_EDGE('',*,*,#3347,.F.);
#4503=ORIENTED_EDGE('',*,*,#3348,.F.);
#4504=ORIENTED_EDGE('',*,*,#3349,.T.);
#4505=ORIENTED_EDGE('',*,*,#3346,.T.);
#4506=ORIENTED_EDGE('',*,*,#3350,.F.);
#4507=ORIENTED_EDGE('',*,*,#3351,.F.);
#4508=ORIENTED_EDGE('',*,*,#3352,.F.);
#4509=ORIENTED_EDGE('',*,*,#3353,.F.);
#4510=ORIENTED_EDGE('',*,*,#3354,.F.);
#4511=ORIENTED_EDGE('',*,*,#3351,.T.);
#4512=ORIENTED_EDGE('',*,*,#3355,.T.);
#4513=ORIENTED_EDGE('',*,*,#3356,.F.);
#4514=ORIENTED_EDGE('',*,*,#3357,.F.);
#4515=ORIENTED_EDGE('',*,*,#3358,.F.);
#4516=ORIENTED_EDGE('',*,*,#3359,.F.);
#4517=ORIENTED_EDGE('',*,*,#3360,.F.);
#4518=ORIENTED_EDGE('',*,*,#3361,.F.);
#4519=ORIENTED_EDGE('',*,*,#3358,.T.);
#4520=ORIENTED_EDGE('',*,*,#3362,.T.);
#4521=ORIENTED_EDGE('',*,*,#3363,.F.);
#4522=ORIENTED_EDGE('',*,*,#3364,.F.);
#4523=ORIENTED_EDGE('',*,*,#3365,.F.);
#4524=ORIENTED_EDGE('',*,*,#3366,.F.);
#4525=ORIENTED_EDGE('',*,*,#3367,.F.);
#4526=ORIENTED_EDGE('',*,*,#3368,.F.);
#4527=ORIENTED_EDGE('',*,*,#3369,.F.);
#4528=ORIENTED_EDGE('',*,*,#3370,.F.);
#4529=ORIENTED_EDGE('',*,*,#3371,.F.);
#4530=ORIENTED_EDGE('',*,*,#3372,.F.);
#4531=ORIENTED_EDGE('',*,*,#3373,.F.);
#4532=ORIENTED_EDGE('',*,*,#3374,.F.);
#4533=ORIENTED_EDGE('',*,*,#3375,.F.);
#4534=ORIENTED_EDGE('',*,*,#3376,.F.);
#4535=ORIENTED_EDGE('',*,*,#3377,.F.);
#4536=ORIENTED_EDGE('',*,*,#3378,.F.);
#4537=ORIENTED_EDGE('',*,*,#3379,.F.);
#4538=ORIENTED_EDGE('',*,*,#3380,.F.);
#4539=ORIENTED_EDGE('',*,*,#3381,.F.);
#4540=ORIENTED_EDGE('',*,*,#3382,.F.);
#4541=ORIENTED_EDGE('',*,*,#3383,.F.);
#4542=ORIENTED_EDGE('',*,*,#3384,.F.);
#4543=ORIENTED_EDGE('',*,*,#3385,.F.);
#4544=ORIENTED_EDGE('',*,*,#3386,.F.);
#4545=ORIENTED_EDGE('',*,*,#3387,.F.);
#4546=ORIENTED_EDGE('',*,*,#3388,.F.);
#4547=ORIENTED_EDGE('',*,*,#3389,.F.);
#4548=ORIENTED_EDGE('',*,*,#3390,.F.);
#4549=ORIENTED_EDGE('',*,*,#3391,.F.);
#4550=ORIENTED_EDGE('',*,*,#3392,.F.);
#4551=ORIENTED_EDGE('',*,*,#3393,.F.);
#4552=ORIENTED_EDGE('',*,*,#3394,.F.);
#4553=ORIENTED_EDGE('',*,*,#3395,.F.);
#4554=ORIENTED_EDGE('',*,*,#3396,.F.);
#4555=ORIENTED_EDGE('',*,*,#3397,.F.);
#4556=ORIENTED_EDGE('',*,*,#3398,.F.);
#4557=ORIENTED_EDGE('',*,*,#3399,.F.);
#4558=ORIENTED_EDGE('',*,*,#3400,.F.);
#4559=ORIENTED_EDGE('',*,*,#3401,.F.);
#4560=ORIENTED_EDGE('',*,*,#3402,.F.);
#4561=ORIENTED_EDGE('',*,*,#3403,.F.);
#4562=ORIENTED_EDGE('',*,*,#3404,.F.);
#4563=ORIENTED_EDGE('',*,*,#3405,.T.);
#4564=ORIENTED_EDGE('',*,*,#3406,.T.);
#4565=ORIENTED_EDGE('',*,*,#3407,.T.);
#4566=ORIENTED_EDGE('',*,*,#3408,.F.);
#4567=ORIENTED_EDGE('',*,*,#3409,.T.);
#4568=ORIENTED_EDGE('',*,*,#3410,.T.);
#4569=ORIENTED_EDGE('',*,*,#3411,.T.);
#4570=ORIENTED_EDGE('',*,*,#3412,.T.);
#4571=ORIENTED_EDGE('',*,*,#3413,.T.);
#4572=ORIENTED_EDGE('',*,*,#3414,.F.);
#4573=ORIENTED_EDGE('',*,*,#3415,.T.);
#4574=ORIENTED_EDGE('',*,*,#3416,.F.);
#4575=ORIENTED_EDGE('',*,*,#3417,.T.);
#4576=ORIENTED_EDGE('',*,*,#3418,.T.);
#4577=ORIENTED_EDGE('',*,*,#3419,.T.);
#4578=ORIENTED_EDGE('',*,*,#3420,.F.);
#4579=ORIENTED_EDGE('',*,*,#3421,.T.);
#4580=ORIENTED_EDGE('',*,*,#3422,.T.);
#4581=ORIENTED_EDGE('',*,*,#3423,.T.);
#4582=ORIENTED_EDGE('',*,*,#3424,.T.);
#4583=ORIENTED_EDGE('',*,*,#3425,.T.);
#4584=ORIENTED_EDGE('',*,*,#3426,.F.);
#4585=ORIENTED_EDGE('',*,*,#3427,.T.);
#4586=ORIENTED_EDGE('',*,*,#3428,.T.);
#4587=ORIENTED_EDGE('',*,*,#3429,.T.);
#4588=ORIENTED_EDGE('',*,*,#3430,.F.);
#4589=ORIENTED_EDGE('',*,*,#3431,.T.);
#4590=ORIENTED_EDGE('',*,*,#3432,.T.);
#4591=ORIENTED_EDGE('',*,*,#3433,.T.);
#4592=ORIENTED_EDGE('',*,*,#3434,.F.);
#4593=ORIENTED_EDGE('',*,*,#3435,.T.);
#4594=ORIENTED_EDGE('',*,*,#3436,.F.);
#4595=ORIENTED_EDGE('',*,*,#3437,.T.);
#4596=ORIENTED_EDGE('',*,*,#3438,.T.);
#4597=ORIENTED_EDGE('',*,*,#3439,.T.);
#4598=ORIENTED_EDGE('',*,*,#3440,.F.);
#4599=ORIENTED_EDGE('',*,*,#3441,.T.);
#4600=ORIENTED_EDGE('',*,*,#3442,.T.);
#4601=ORIENTED_EDGE('',*,*,#3443,.T.);
#4602=ORIENTED_EDGE('',*,*,#3444,.T.);
#4603=ORIENTED_EDGE('',*,*,#3445,.T.);
#4604=ORIENTED_EDGE('',*,*,#3446,.F.);
#4605=ORIENTED_EDGE('',*,*,#3447,.T.);
#4606=ORIENTED_EDGE('',*,*,#3448,.T.);
#4607=ORIENTED_EDGE('',*,*,#3449,.T.);
#4608=ORIENTED_EDGE('',*,*,#3450,.F.);
#4609=ORIENTED_EDGE('',*,*,#3451,.T.);
#4610=ORIENTED_EDGE('',*,*,#3452,.T.);
#4611=ORIENTED_EDGE('',*,*,#3453,.T.);
#4612=ORIENTED_EDGE('',*,*,#3454,.F.);
#4613=ORIENTED_EDGE('',*,*,#3455,.T.);
#4614=ORIENTED_EDGE('',*,*,#3456,.T.);
#4615=ORIENTED_EDGE('',*,*,#3457,.T.);
#4616=ORIENTED_EDGE('',*,*,#3458,.F.);
#4617=ORIENTED_EDGE('',*,*,#3459,.T.);
#4618=ORIENTED_EDGE('',*,*,#3460,.T.);
#4619=ORIENTED_EDGE('',*,*,#3461,.T.);
#4620=ORIENTED_EDGE('',*,*,#3462,.F.);
#4621=ORIENTED_EDGE('',*,*,#3341,.T.);
#4622=ORIENTED_EDGE('',*,*,#3463,.T.);
#4623=ORIENTED_EDGE('',*,*,#3464,.T.);
#4624=ORIENTED_EDGE('',*,*,#3465,.F.);
#4625=ORIENTED_EDGE('',*,*,#3348,.T.);
#4626=ORIENTED_EDGE('',*,*,#3466,.F.);
#4627=ORIENTED_EDGE('',*,*,#3467,.T.);
#4628=ORIENTED_EDGE('',*,*,#3468,.T.);
#4629=ORIENTED_EDGE('',*,*,#3363,.T.);
#4630=ORIENTED_EDGE('',*,*,#3469,.F.);
#4631=ORIENTED_EDGE('',*,*,#3470,.T.);
#4632=ORIENTED_EDGE('',*,*,#3471,.T.);
#4633=ORIENTED_EDGE('',*,*,#3472,.T.);
#4634=ORIENTED_EDGE('',*,*,#3473,.F.);
#4635=ORIENTED_EDGE('',*,*,#3474,.T.);
#4636=ORIENTED_EDGE('',*,*,#3475,.T.);
#4637=ORIENTED_EDGE('',*,*,#3476,.T.);
#4638=ORIENTED_EDGE('',*,*,#3477,.T.);
#4639=ORIENTED_EDGE('',*,*,#3478,.T.);
#4640=ORIENTED_EDGE('',*,*,#3479,.F.);
#4641=ORIENTED_EDGE('',*,*,#3480,.T.);
#4642=ORIENTED_EDGE('',*,*,#3481,.F.);
#4643=ORIENTED_EDGE('',*,*,#3482,.T.);
#4644=ORIENTED_EDGE('',*,*,#3483,.T.);
#4645=ORIENTED_EDGE('',*,*,#3484,.T.);
#4646=ORIENTED_EDGE('',*,*,#3485,.F.);
#4647=ORIENTED_EDGE('',*,*,#3486,.T.);
#4648=ORIENTED_EDGE('',*,*,#3487,.T.);
#4649=ORIENTED_EDGE('',*,*,#3488,.T.);
#4650=ORIENTED_EDGE('',*,*,#3489,.F.);
#4651=ORIENTED_EDGE('',*,*,#3490,.T.);
#4652=ORIENTED_EDGE('',*,*,#3491,.T.);
#4653=ORIENTED_EDGE('',*,*,#3492,.T.);
#4654=ORIENTED_EDGE('',*,*,#3493,.F.);
#4655=ORIENTED_EDGE('',*,*,#3494,.T.);
#4656=ORIENTED_EDGE('',*,*,#3495,.T.);
#4657=ORIENTED_EDGE('',*,*,#3496,.T.);
#4658=ORIENTED_EDGE('',*,*,#3497,.F.);
#4659=ORIENTED_EDGE('',*,*,#3498,.T.);
#4660=ORIENTED_EDGE('',*,*,#3499,.T.);
#4661=ORIENTED_EDGE('',*,*,#3500,.T.);
#4662=ORIENTED_EDGE('',*,*,#3501,.T.);
#4663=ORIENTED_EDGE('',*,*,#3502,.T.);
#4664=ORIENTED_EDGE('',*,*,#3503,.F.);
#4665=ORIENTED_EDGE('',*,*,#3504,.T.);
#4666=ORIENTED_EDGE('',*,*,#3505,.T.);
#4667=ORIENTED_EDGE('',*,*,#3506,.T.);
#4668=ORIENTED_EDGE('',*,*,#3507,.F.);
#4669=ORIENTED_EDGE('',*,*,#3508,.T.);
#4670=ORIENTED_EDGE('',*,*,#3509,.T.);
#4671=ORIENTED_EDGE('',*,*,#3510,.T.);
#4672=ORIENTED_EDGE('',*,*,#3511,.F.);
#4673=ORIENTED_EDGE('',*,*,#3512,.T.);
#4674=ORIENTED_EDGE('',*,*,#3513,.F.);
#4675=ORIENTED_EDGE('',*,*,#3514,.T.);
#4676=ORIENTED_EDGE('',*,*,#3515,.T.);
#4677=ORIENTED_EDGE('',*,*,#3516,.T.);
#4678=ORIENTED_EDGE('',*,*,#3410,.F.);
#4679=ORIENTED_EDGE('',*,*,#3517,.T.);
#4680=ORIENTED_EDGE('',*,*,#3518,.T.);
#4681=ORIENTED_EDGE('',*,*,#3519,.T.);
#4682=ORIENTED_EDGE('',*,*,#3520,.T.);
#4683=ORIENTED_EDGE('',*,*,#3521,.T.);
#4684=ORIENTED_EDGE('',*,*,#3412,.F.);
#4685=ORIENTED_EDGE('',*,*,#3522,.T.);
#4686=ORIENTED_EDGE('',*,*,#3523,.T.);
#4687=ORIENTED_EDGE('',*,*,#3524,.T.);
#4688=ORIENTED_EDGE('',*,*,#3525,.T.);
#4689=ORIENTED_EDGE('',*,*,#3526,.T.);
#4690=ORIENTED_EDGE('',*,*,#3424,.F.);
#4691=ORIENTED_EDGE('',*,*,#3527,.T.);
#4692=ORIENTED_EDGE('',*,*,#3528,.T.);
#4693=ORIENTED_EDGE('',*,*,#3529,.T.);
#4694=ORIENTED_EDGE('',*,*,#3530,.T.);
#4695=ORIENTED_EDGE('',*,*,#3531,.T.);
#4696=ORIENTED_EDGE('',*,*,#3428,.F.);
#4697=ORIENTED_EDGE('',*,*,#3532,.T.);
#4698=ORIENTED_EDGE('',*,*,#3533,.T.);
#4699=ORIENTED_EDGE('',*,*,#3534,.T.);
#4700=ORIENTED_EDGE('',*,*,#3535,.T.);
#4701=ORIENTED_EDGE('',*,*,#3536,.T.);
#4702=ORIENTED_EDGE('',*,*,#3406,.F.);
#4703=ORIENTED_EDGE('',*,*,#3537,.T.);
#4704=ORIENTED_EDGE('',*,*,#3538,.T.);
#4705=ORIENTED_EDGE('',*,*,#3539,.T.);
#4706=ORIENTED_EDGE('',*,*,#3540,.T.);
#4707=ORIENTED_EDGE('',*,*,#3541,.T.);
#4708=ORIENTED_EDGE('',*,*,#3432,.F.);
#4709=ORIENTED_EDGE('',*,*,#3542,.T.);
#4710=ORIENTED_EDGE('',*,*,#3543,.T.);
#4711=ORIENTED_EDGE('',*,*,#3544,.T.);
#4712=ORIENTED_EDGE('',*,*,#3545,.T.);
#4713=ORIENTED_EDGE('',*,*,#3546,.T.);
#4714=ORIENTED_EDGE('',*,*,#3444,.F.);
#4715=ORIENTED_EDGE('',*,*,#3547,.T.);
#4716=ORIENTED_EDGE('',*,*,#3548,.T.);
#4717=ORIENTED_EDGE('',*,*,#3549,.T.);
#4718=ORIENTED_EDGE('',*,*,#3550,.T.);
#4719=ORIENTED_EDGE('',*,*,#3551,.T.);
#4720=ORIENTED_EDGE('',*,*,#3448,.F.);
#4721=ORIENTED_EDGE('',*,*,#3552,.T.);
#4722=ORIENTED_EDGE('',*,*,#3553,.T.);
#4723=ORIENTED_EDGE('',*,*,#3554,.T.);
#4724=ORIENTED_EDGE('',*,*,#3555,.T.);
#4725=ORIENTED_EDGE('',*,*,#3556,.T.);
#4726=ORIENTED_EDGE('',*,*,#3442,.F.);
#4727=ORIENTED_EDGE('',*,*,#3557,.T.);
#4728=ORIENTED_EDGE('',*,*,#3558,.T.);
#4729=ORIENTED_EDGE('',*,*,#3559,.T.);
#4730=ORIENTED_EDGE('',*,*,#3560,.T.);
#4731=ORIENTED_EDGE('',*,*,#3561,.T.);
#4732=ORIENTED_EDGE('',*,*,#3438,.F.);
#4733=ORIENTED_EDGE('',*,*,#3562,.T.);
#4734=ORIENTED_EDGE('',*,*,#3563,.T.);
#4735=ORIENTED_EDGE('',*,*,#3564,.T.);
#4736=ORIENTED_EDGE('',*,*,#3565,.T.);
#4737=ORIENTED_EDGE('',*,*,#3566,.T.);
#4738=ORIENTED_EDGE('',*,*,#3452,.F.);
#4739=ORIENTED_EDGE('',*,*,#3567,.T.);
#4740=ORIENTED_EDGE('',*,*,#3568,.T.);
#4741=ORIENTED_EDGE('',*,*,#3569,.T.);
#4742=ORIENTED_EDGE('',*,*,#3570,.T.);
#4743=ORIENTED_EDGE('',*,*,#3571,.T.);
#4744=ORIENTED_EDGE('',*,*,#3456,.F.);
#4745=ORIENTED_EDGE('',*,*,#3572,.T.);
#4746=ORIENTED_EDGE('',*,*,#3573,.T.);
#4747=ORIENTED_EDGE('',*,*,#3574,.T.);
#4748=ORIENTED_EDGE('',*,*,#3575,.T.);
#4749=ORIENTED_EDGE('',*,*,#3576,.T.);
#4750=ORIENTED_EDGE('',*,*,#3460,.F.);
#4751=ORIENTED_EDGE('',*,*,#3340,.T.);
#4752=ORIENTED_EDGE('',*,*,#3338,.T.);
#4753=ORIENTED_EDGE('',*,*,#3577,.T.);
#4754=ORIENTED_EDGE('',*,*,#3578,.T.);
#4755=ORIENTED_EDGE('',*,*,#3579,.T.);
#4756=ORIENTED_EDGE('',*,*,#3463,.F.);
#4757=ORIENTED_EDGE('',*,*,#3347,.T.);
#4758=ORIENTED_EDGE('',*,*,#3345,.T.);
#4759=ORIENTED_EDGE('',*,*,#3580,.T.);
#4760=ORIENTED_EDGE('',*,*,#3581,.T.);
#4761=ORIENTED_EDGE('',*,*,#3582,.T.);
#4762=ORIENTED_EDGE('',*,*,#3501,.F.);
#4763=ORIENTED_EDGE('',*,*,#3583,.T.);
#4764=ORIENTED_EDGE('',*,*,#3394,.T.);
#4765=ORIENTED_EDGE('',*,*,#3584,.T.);
#4766=ORIENTED_EDGE('',*,*,#3585,.T.);
#4767=ORIENTED_EDGE('',*,*,#3586,.T.);
#4768=ORIENTED_EDGE('',*,*,#3499,.F.);
#4769=ORIENTED_EDGE('',*,*,#3587,.T.);
#4770=ORIENTED_EDGE('',*,*,#3390,.T.);
#4771=ORIENTED_EDGE('',*,*,#3588,.T.);
#4772=ORIENTED_EDGE('',*,*,#3589,.T.);
#4773=ORIENTED_EDGE('',*,*,#3590,.T.);
#4774=ORIENTED_EDGE('',*,*,#3505,.F.);
#4775=ORIENTED_EDGE('',*,*,#3591,.T.);
#4776=ORIENTED_EDGE('',*,*,#3398,.T.);
#4777=ORIENTED_EDGE('',*,*,#3592,.T.);
#4778=ORIENTED_EDGE('',*,*,#3593,.T.);
#4779=ORIENTED_EDGE('',*,*,#3594,.T.);
#4780=ORIENTED_EDGE('',*,*,#3509,.F.);
#4781=ORIENTED_EDGE('',*,*,#3595,.T.);
#4782=ORIENTED_EDGE('',*,*,#3402,.T.);
#4783=ORIENTED_EDGE('',*,*,#3596,.T.);
#4784=ORIENTED_EDGE('',*,*,#3597,.T.);
#4785=ORIENTED_EDGE('',*,*,#3598,.T.);
#4786=ORIENTED_EDGE('',*,*,#3495,.F.);
#4787=ORIENTED_EDGE('',*,*,#3599,.T.);
#4788=ORIENTED_EDGE('',*,*,#3386,.T.);
#4789=ORIENTED_EDGE('',*,*,#3600,.T.);
#4790=ORIENTED_EDGE('',*,*,#3601,.T.);
#4791=ORIENTED_EDGE('',*,*,#3602,.T.);
#4792=ORIENTED_EDGE('',*,*,#3491,.F.);
#4793=ORIENTED_EDGE('',*,*,#3603,.T.);
#4794=ORIENTED_EDGE('',*,*,#3604,.T.);
#4795=ORIENTED_EDGE('',*,*,#3605,.T.);
#4796=ORIENTED_EDGE('',*,*,#3382,.T.);
#4797=ORIENTED_EDGE('',*,*,#3606,.T.);
#4798=ORIENTED_EDGE('',*,*,#3487,.F.);
#4799=ORIENTED_EDGE('',*,*,#3607,.T.);
#4800=ORIENTED_EDGE('',*,*,#3608,.T.);
#4801=ORIENTED_EDGE('',*,*,#3609,.T.);
#4802=ORIENTED_EDGE('',*,*,#3378,.T.);
#4803=ORIENTED_EDGE('',*,*,#3610,.T.);
#4804=ORIENTED_EDGE('',*,*,#3483,.F.);
#4805=ORIENTED_EDGE('',*,*,#3611,.T.);
#4806=ORIENTED_EDGE('',*,*,#3612,.T.);
#4807=ORIENTED_EDGE('',*,*,#3613,.T.);
#4808=ORIENTED_EDGE('',*,*,#3374,.T.);
#4809=ORIENTED_EDGE('',*,*,#3614,.T.);
#4810=ORIENTED_EDGE('',*,*,#3475,.F.);
#4811=ORIENTED_EDGE('',*,*,#3615,.T.);
#4812=ORIENTED_EDGE('',*,*,#3616,.T.);
#4813=ORIENTED_EDGE('',*,*,#3617,.T.);
#4814=ORIENTED_EDGE('',*,*,#3366,.T.);
#4815=ORIENTED_EDGE('',*,*,#3618,.T.);
#4816=ORIENTED_EDGE('',*,*,#3477,.F.);
#4817=ORIENTED_EDGE('',*,*,#3619,.T.);
#4818=ORIENTED_EDGE('',*,*,#3620,.T.);
#4819=ORIENTED_EDGE('',*,*,#3621,.T.);
#4820=ORIENTED_EDGE('',*,*,#3370,.T.);
#4821=ORIENTED_EDGE('',*,*,#3622,.T.);
#4822=ORIENTED_EDGE('',*,*,#3471,.F.);
#4823=ORIENTED_EDGE('',*,*,#3623,.T.);
#4824=ORIENTED_EDGE('',*,*,#3624,.T.);
#4825=ORIENTED_EDGE('',*,*,#3625,.T.);
#4826=ORIENTED_EDGE('',*,*,#3359,.T.);
#4827=ORIENTED_EDGE('',*,*,#3361,.T.);
#4828=ORIENTED_EDGE('',*,*,#3468,.F.);
#4829=ORIENTED_EDGE('',*,*,#3626,.T.);
#4830=ORIENTED_EDGE('',*,*,#3627,.T.);
#4831=ORIENTED_EDGE('',*,*,#3628,.T.);
#4832=ORIENTED_EDGE('',*,*,#3352,.T.);
#4833=ORIENTED_EDGE('',*,*,#3354,.T.);
#4834=ORIENTED_EDGE('',*,*,#3629,.F.);
#4835=ORIENTED_EDGE('',*,*,#3630,.T.);
#4836=ORIENTED_EDGE('',*,*,#3631,.T.);
#4837=ORIENTED_EDGE('',*,*,#3632,.T.);
#4838=ORIENTED_EDGE('',*,*,#3633,.T.);
#4839=ORIENTED_EDGE('',*,*,#3634,.T.);
#4840=ORIENTED_EDGE('',*,*,#3515,.F.);
#4841=ORIENTED_EDGE('',*,*,#3635,.T.);
#4842=ORIENTED_EDGE('',*,*,#3636,.T.);
#4843=ORIENTED_EDGE('',*,*,#3637,.T.);
#4844=ORIENTED_EDGE('',*,*,#3638,.T.);
#4845=ORIENTED_EDGE('',*,*,#3639,.T.);
#4846=ORIENTED_EDGE('',*,*,#3422,.F.);
#4847=ORIENTED_EDGE('',*,*,#3640,.T.);
#4848=ORIENTED_EDGE('',*,*,#3641,.T.);
#4849=ORIENTED_EDGE('',*,*,#3642,.T.);
#4850=ORIENTED_EDGE('',*,*,#3643,.T.);
#4851=ORIENTED_EDGE('',*,*,#3644,.T.);
#4852=ORIENTED_EDGE('',*,*,#3418,.F.);
#4853=ORIENTED_EDGE('',*,*,#3645,.T.);
#4854=ORIENTED_EDGE('',*,*,#3646,.T.);
#4855=ORIENTED_EDGE('',*,*,#3647,.T.);
#4856=ORIENTED_EDGE('',*,*,#3648,.T.);
#4857=ORIENTED_EDGE('',*,*,#3649,.T.);
#4858=ORIENTED_EDGE('',*,*,#3650,.T.);
#4859=ORIENTED_EDGE('',*,*,#3332,.T.);
#4860=ORIENTED_EDGE('',*,*,#3651,.T.);
#4861=ORIENTED_EDGE('',*,*,#3652,.T.);
#4862=ORIENTED_EDGE('',*,*,#3653,.F.);
#4863=ORIENTED_EDGE('',*,*,#3408,.T.);
#4864=ORIENTED_EDGE('',*,*,#3654,.F.);
#4865=ORIENTED_EDGE('',*,*,#3655,.T.);
#4866=ORIENTED_EDGE('',*,*,#3656,.F.);
#4867=ORIENTED_EDGE('',*,*,#3657,.T.);
#4868=ORIENTED_EDGE('',*,*,#3658,.F.);
#4869=ORIENTED_EDGE('',*,*,#3416,.T.);
#4870=ORIENTED_EDGE('',*,*,#3659,.F.);
#4871=ORIENTED_EDGE('',*,*,#3660,.T.);
#4872=ORIENTED_EDGE('',*,*,#3661,.F.);
#4873=ORIENTED_EDGE('',*,*,#3662,.T.);
#4874=ORIENTED_EDGE('',*,*,#3663,.F.);
#4875=ORIENTED_EDGE('',*,*,#3420,.T.);
#4876=ORIENTED_EDGE('',*,*,#3664,.F.);
#4877=ORIENTED_EDGE('',*,*,#3665,.T.);
#4878=ORIENTED_EDGE('',*,*,#3666,.F.);
#4879=ORIENTED_EDGE('',*,*,#3667,.T.);
#4880=ORIENTED_EDGE('',*,*,#3668,.F.);
#4881=ORIENTED_EDGE('',*,*,#3513,.T.);
#4882=ORIENTED_EDGE('',*,*,#3669,.F.);
#4883=ORIENTED_EDGE('',*,*,#3670,.T.);
#4884=ORIENTED_EDGE('',*,*,#3671,.F.);
#4885=ORIENTED_EDGE('',*,*,#3672,.T.);
#4886=ORIENTED_EDGE('',*,*,#3673,.F.);
#4887=ORIENTED_EDGE('',*,*,#3674,.T.);
#4888=ORIENTED_EDGE('',*,*,#3355,.F.);
#4889=ORIENTED_EDGE('',*,*,#3350,.T.);
#4890=ORIENTED_EDGE('',*,*,#3675,.F.);
#4891=ORIENTED_EDGE('',*,*,#3676,.T.);
#4892=ORIENTED_EDGE('',*,*,#3677,.F.);
#4893=ORIENTED_EDGE('',*,*,#3466,.T.);
#4894=ORIENTED_EDGE('',*,*,#3362,.F.);
#4895=ORIENTED_EDGE('',*,*,#3357,.T.);
#4896=ORIENTED_EDGE('',*,*,#3678,.F.);
#4897=ORIENTED_EDGE('',*,*,#3679,.T.);
#4898=ORIENTED_EDGE('',*,*,#3680,.F.);
#4899=ORIENTED_EDGE('',*,*,#3469,.T.);
#4900=ORIENTED_EDGE('',*,*,#3681,.F.);
#4901=ORIENTED_EDGE('',*,*,#3368,.T.);
#4902=ORIENTED_EDGE('',*,*,#3682,.F.);
#4903=ORIENTED_EDGE('',*,*,#3683,.T.);
#4904=ORIENTED_EDGE('',*,*,#3684,.F.);
#4905=ORIENTED_EDGE('',*,*,#3479,.T.);
#4906=ORIENTED_EDGE('',*,*,#3685,.F.);
#4907=ORIENTED_EDGE('',*,*,#3364,.T.);
#4908=ORIENTED_EDGE('',*,*,#3686,.F.);
#4909=ORIENTED_EDGE('',*,*,#3687,.T.);
#4910=ORIENTED_EDGE('',*,*,#3688,.F.);
#4911=ORIENTED_EDGE('',*,*,#3473,.T.);
#4912=ORIENTED_EDGE('',*,*,#3689,.F.);
#4913=ORIENTED_EDGE('',*,*,#3372,.T.);
#4914=ORIENTED_EDGE('',*,*,#3690,.F.);
#4915=ORIENTED_EDGE('',*,*,#3691,.T.);
#4916=ORIENTED_EDGE('',*,*,#3692,.F.);
#4917=ORIENTED_EDGE('',*,*,#3481,.T.);
#4918=ORIENTED_EDGE('',*,*,#3693,.F.);
#4919=ORIENTED_EDGE('',*,*,#3376,.T.);
#4920=ORIENTED_EDGE('',*,*,#3694,.F.);
#4921=ORIENTED_EDGE('',*,*,#3695,.T.);
#4922=ORIENTED_EDGE('',*,*,#3696,.F.);
#4923=ORIENTED_EDGE('',*,*,#3485,.T.);
#4924=ORIENTED_EDGE('',*,*,#3697,.F.);
#4925=ORIENTED_EDGE('',*,*,#3380,.T.);
#4926=ORIENTED_EDGE('',*,*,#3698,.F.);
#4927=ORIENTED_EDGE('',*,*,#3699,.T.);
#4928=ORIENTED_EDGE('',*,*,#3700,.F.);
#4929=ORIENTED_EDGE('',*,*,#3489,.T.);
#4930=ORIENTED_EDGE('',*,*,#3701,.F.);
#4931=ORIENTED_EDGE('',*,*,#3702,.T.);
#4932=ORIENTED_EDGE('',*,*,#3703,.F.);
#4933=ORIENTED_EDGE('',*,*,#3384,.T.);
#4934=ORIENTED_EDGE('',*,*,#3704,.F.);
#4935=ORIENTED_EDGE('',*,*,#3493,.T.);
#4936=ORIENTED_EDGE('',*,*,#3705,.F.);
#4937=ORIENTED_EDGE('',*,*,#3706,.T.);
#4938=ORIENTED_EDGE('',*,*,#3707,.F.);
#4939=ORIENTED_EDGE('',*,*,#3400,.T.);
#4940=ORIENTED_EDGE('',*,*,#3708,.F.);
#4941=ORIENTED_EDGE('',*,*,#3511,.T.);
#4942=ORIENTED_EDGE('',*,*,#3709,.F.);
#4943=ORIENTED_EDGE('',*,*,#3710,.T.);
#4944=ORIENTED_EDGE('',*,*,#3711,.F.);
#4945=ORIENTED_EDGE('',*,*,#3396,.T.);
#4946=ORIENTED_EDGE('',*,*,#3712,.F.);
#4947=ORIENTED_EDGE('',*,*,#3507,.T.);
#4948=ORIENTED_EDGE('',*,*,#3713,.F.);
#4949=ORIENTED_EDGE('',*,*,#3714,.T.);
#4950=ORIENTED_EDGE('',*,*,#3715,.F.);
#4951=ORIENTED_EDGE('',*,*,#3388,.T.);
#4952=ORIENTED_EDGE('',*,*,#3716,.F.);
#4953=ORIENTED_EDGE('',*,*,#3497,.T.);
#4954=ORIENTED_EDGE('',*,*,#3717,.F.);
#4955=ORIENTED_EDGE('',*,*,#3718,.T.);
#4956=ORIENTED_EDGE('',*,*,#3719,.F.);
#4957=ORIENTED_EDGE('',*,*,#3392,.T.);
#4958=ORIENTED_EDGE('',*,*,#3720,.F.);
#4959=ORIENTED_EDGE('',*,*,#3503,.T.);
#4960=ORIENTED_EDGE('',*,*,#3721,.F.);
#4961=ORIENTED_EDGE('',*,*,#3722,.T.);
#4962=ORIENTED_EDGE('',*,*,#3723,.F.);
#4963=ORIENTED_EDGE('',*,*,#3343,.T.);
#4964=ORIENTED_EDGE('',*,*,#3349,.F.);
#4965=ORIENTED_EDGE('',*,*,#3465,.T.);
#4966=ORIENTED_EDGE('',*,*,#3724,.F.);
#4967=ORIENTED_EDGE('',*,*,#3725,.T.);
#4968=ORIENTED_EDGE('',*,*,#3726,.F.);
#4969=ORIENTED_EDGE('',*,*,#3336,.T.);
#4970=ORIENTED_EDGE('',*,*,#3342,.F.);
#4971=ORIENTED_EDGE('',*,*,#3462,.T.);
#4972=ORIENTED_EDGE('',*,*,#3727,.F.);
#4973=ORIENTED_EDGE('',*,*,#3728,.T.);
#4974=ORIENTED_EDGE('',*,*,#3729,.F.);
#4975=ORIENTED_EDGE('',*,*,#3730,.T.);
#4976=ORIENTED_EDGE('',*,*,#3731,.F.);
#4977=ORIENTED_EDGE('',*,*,#3458,.T.);
#4978=ORIENTED_EDGE('',*,*,#3732,.F.);
#4979=ORIENTED_EDGE('',*,*,#3733,.T.);
#4980=ORIENTED_EDGE('',*,*,#3734,.F.);
#4981=ORIENTED_EDGE('',*,*,#3735,.T.);
#4982=ORIENTED_EDGE('',*,*,#3736,.F.);
#4983=ORIENTED_EDGE('',*,*,#3454,.T.);
#4984=ORIENTED_EDGE('',*,*,#3737,.F.);
#4985=ORIENTED_EDGE('',*,*,#3738,.T.);
#4986=ORIENTED_EDGE('',*,*,#3739,.F.);
#4987=ORIENTED_EDGE('',*,*,#3740,.T.);
#4988=ORIENTED_EDGE('',*,*,#3741,.F.);
#4989=ORIENTED_EDGE('',*,*,#3436,.T.);
#4990=ORIENTED_EDGE('',*,*,#3742,.F.);
#4991=ORIENTED_EDGE('',*,*,#3743,.T.);
#4992=ORIENTED_EDGE('',*,*,#3744,.F.);
#4993=ORIENTED_EDGE('',*,*,#3745,.T.);
#4994=ORIENTED_EDGE('',*,*,#3746,.F.);
#4995=ORIENTED_EDGE('',*,*,#3440,.T.);
#4996=ORIENTED_EDGE('',*,*,#3747,.F.);
#4997=ORIENTED_EDGE('',*,*,#3748,.T.);
#4998=ORIENTED_EDGE('',*,*,#3749,.F.);
#4999=ORIENTED_EDGE('',*,*,#3750,.T.);
#5000=ORIENTED_EDGE('',*,*,#3751,.F.);
#5001=ORIENTED_EDGE('',*,*,#3450,.T.);
#5002=ORIENTED_EDGE('',*,*,#3752,.F.);
#5003=ORIENTED_EDGE('',*,*,#3753,.T.);
#5004=ORIENTED_EDGE('',*,*,#3754,.F.);
#5005=ORIENTED_EDGE('',*,*,#3755,.T.);
#5006=ORIENTED_EDGE('',*,*,#3756,.F.);
#5007=ORIENTED_EDGE('',*,*,#3446,.T.);
#5008=ORIENTED_EDGE('',*,*,#3757,.F.);
#5009=ORIENTED_EDGE('',*,*,#3758,.T.);
#5010=ORIENTED_EDGE('',*,*,#3759,.F.);
#5011=ORIENTED_EDGE('',*,*,#3760,.T.);
#5012=ORIENTED_EDGE('',*,*,#3761,.F.);
#5013=ORIENTED_EDGE('',*,*,#3434,.T.);
#5014=ORIENTED_EDGE('',*,*,#3762,.F.);
#5015=ORIENTED_EDGE('',*,*,#3763,.T.);
#5016=ORIENTED_EDGE('',*,*,#3764,.F.);
#5017=ORIENTED_EDGE('',*,*,#3765,.T.);
#5018=ORIENTED_EDGE('',*,*,#3766,.F.);
#5019=ORIENTED_EDGE('',*,*,#3404,.T.);
#5020=ORIENTED_EDGE('',*,*,#3767,.F.);
#5021=ORIENTED_EDGE('',*,*,#3768,.T.);
#5022=ORIENTED_EDGE('',*,*,#3769,.F.);
#5023=ORIENTED_EDGE('',*,*,#3770,.T.);
#5024=ORIENTED_EDGE('',*,*,#3771,.F.);
#5025=ORIENTED_EDGE('',*,*,#3430,.T.);
#5026=ORIENTED_EDGE('',*,*,#3772,.F.);
#5027=ORIENTED_EDGE('',*,*,#3773,.T.);
#5028=ORIENTED_EDGE('',*,*,#3774,.F.);
#5029=ORIENTED_EDGE('',*,*,#3775,.T.);
#5030=ORIENTED_EDGE('',*,*,#3776,.F.);
#5031=ORIENTED_EDGE('',*,*,#3426,.T.);
#5032=ORIENTED_EDGE('',*,*,#3777,.F.);
#5033=ORIENTED_EDGE('',*,*,#3778,.T.);
#5034=ORIENTED_EDGE('',*,*,#3779,.F.);
#5035=ORIENTED_EDGE('',*,*,#3780,.T.);
#5036=ORIENTED_EDGE('',*,*,#3781,.F.);
#5037=ORIENTED_EDGE('',*,*,#3414,.T.);
#5038=ORIENTED_EDGE('',*,*,#3782,.F.);
#5039=ORIENTED_EDGE('',*,*,#3783,.T.);
#5040=ORIENTED_EDGE('',*,*,#3784,.F.);
#5041=ORIENTED_EDGE('',*,*,#3785,.T.);
#5042=ORIENTED_EDGE('',*,*,#3334,.F.);
#5043=ORIENTED_EDGE('',*,*,#3786,.F.);
#5044=ORIENTED_EDGE('',*,*,#3787,.F.);
#5045=ORIENTED_EDGE('',*,*,#3788,.F.);
#5046=ORIENTED_EDGE('',*,*,#3629,.T.);
#5047=ORIENTED_EDGE('',*,*,#3356,.T.);
#5048=ORIENTED_EDGE('',*,*,#3674,.F.);
#5049=ORIENTED_EDGE('',*,*,#3789,.T.);
#5050=ORIENTED_EDGE('',*,*,#3634,.F.);
#5051=ORIENTED_EDGE('',*,*,#3790,.T.);
#5052=ORIENTED_EDGE('',*,*,#3669,.T.);
#5053=ORIENTED_EDGE('',*,*,#3516,.F.);
#5054=ORIENTED_EDGE('',*,*,#3673,.T.);
#5055=ORIENTED_EDGE('',*,*,#3791,.T.);
#5056=ORIENTED_EDGE('',*,*,#3630,.F.);
#5057=ORIENTED_EDGE('',*,*,#3789,.F.);
#5058=ORIENTED_EDGE('',*,*,#3671,.T.);
#5059=ORIENTED_EDGE('',*,*,#3792,.T.);
#5060=ORIENTED_EDGE('',*,*,#3632,.F.);
#5061=ORIENTED_EDGE('',*,*,#3793,.T.);
#5062=ORIENTED_EDGE('',*,*,#3633,.F.);
#5063=ORIENTED_EDGE('',*,*,#3792,.F.);
#5064=ORIENTED_EDGE('',*,*,#3670,.F.);
#5065=ORIENTED_EDGE('',*,*,#3790,.F.);
#5066=ORIENTED_EDGE('',*,*,#3631,.F.);
#5067=ORIENTED_EDGE('',*,*,#3791,.F.);
#5068=ORIENTED_EDGE('',*,*,#3672,.F.);
#5069=ORIENTED_EDGE('',*,*,#3793,.F.);
#5070=ORIENTED_EDGE('',*,*,#3668,.T.);
#5071=ORIENTED_EDGE('',*,*,#3794,.T.);
#5072=ORIENTED_EDGE('',*,*,#3635,.F.);
#5073=ORIENTED_EDGE('',*,*,#3514,.F.);
#5074=ORIENTED_EDGE('',*,*,#3639,.F.);
#5075=ORIENTED_EDGE('',*,*,#3795,.T.);
#5076=ORIENTED_EDGE('',*,*,#3664,.T.);
#5077=ORIENTED_EDGE('',*,*,#3423,.F.);
#5078=ORIENTED_EDGE('',*,*,#3638,.F.);
#5079=ORIENTED_EDGE('',*,*,#3796,.F.);
#5080=ORIENTED_EDGE('',*,*,#3665,.F.);
#5081=ORIENTED_EDGE('',*,*,#3795,.F.);
#5082=ORIENTED_EDGE('',*,*,#3666,.T.);
#5083=ORIENTED_EDGE('',*,*,#3796,.T.);
#5084=ORIENTED_EDGE('',*,*,#3637,.F.);
#5085=ORIENTED_EDGE('',*,*,#3797,.T.);
#5086=ORIENTED_EDGE('',*,*,#3636,.F.);
#5087=ORIENTED_EDGE('',*,*,#3794,.F.);
#5088=ORIENTED_EDGE('',*,*,#3667,.F.);
#5089=ORIENTED_EDGE('',*,*,#3797,.F.);
#5090=ORIENTED_EDGE('',*,*,#3708,.T.);
#5091=ORIENTED_EDGE('',*,*,#3403,.T.);
#5092=ORIENTED_EDGE('',*,*,#3595,.F.);
#5093=ORIENTED_EDGE('',*,*,#3512,.F.);
#5094=ORIENTED_EDGE('',*,*,#3598,.F.);
#5095=ORIENTED_EDGE('',*,*,#3798,.T.);
#5096=ORIENTED_EDGE('',*,*,#3705,.T.);
#5097=ORIENTED_EDGE('',*,*,#3496,.F.);
#5098=ORIENTED_EDGE('',*,*,#3597,.F.);
#5099=ORIENTED_EDGE('',*,*,#3799,.F.);
#5100=ORIENTED_EDGE('',*,*,#3706,.F.);
#5101=ORIENTED_EDGE('',*,*,#3798,.F.);
#5102=ORIENTED_EDGE('',*,*,#3707,.T.);
#5103=ORIENTED_EDGE('',*,*,#3799,.T.);
#5104=ORIENTED_EDGE('',*,*,#3596,.F.);
#5105=ORIENTED_EDGE('',*,*,#3401,.T.);
#5106=ORIENTED_EDGE('',*,*,#3712,.T.);
#5107=ORIENTED_EDGE('',*,*,#3399,.T.);
#5108=ORIENTED_EDGE('',*,*,#3591,.F.);
#5109=ORIENTED_EDGE('',*,*,#3508,.F.);
#5110=ORIENTED_EDGE('',*,*,#3594,.F.);
#5111=ORIENTED_EDGE('',*,*,#3800,.T.);
#5112=ORIENTED_EDGE('',*,*,#3709,.T.);
#5113=ORIENTED_EDGE('',*,*,#3510,.F.);
#5114=ORIENTED_EDGE('',*,*,#3593,.F.);
#5115=ORIENTED_EDGE('',*,*,#3801,.F.);
#5116=ORIENTED_EDGE('',*,*,#3710,.F.);
#5117=ORIENTED_EDGE('',*,*,#3800,.F.);
#5118=ORIENTED_EDGE('',*,*,#3711,.T.);
#5119=ORIENTED_EDGE('',*,*,#3801,.T.);
#5120=ORIENTED_EDGE('',*,*,#3592,.F.);
#5121=ORIENTED_EDGE('',*,*,#3397,.T.);
#5122=ORIENTED_EDGE('',*,*,#3720,.T.);
#5123=ORIENTED_EDGE('',*,*,#3395,.T.);
#5124=ORIENTED_EDGE('',*,*,#3583,.F.);
#5125=ORIENTED_EDGE('',*,*,#3504,.F.);
#5126=ORIENTED_EDGE('',*,*,#3586,.F.);
#5127=ORIENTED_EDGE('',*,*,#3802,.T.);
#5128=ORIENTED_EDGE('',*,*,#3717,.T.);
#5129=ORIENTED_EDGE('',*,*,#3500,.F.);
#5130=ORIENTED_EDGE('',*,*,#3585,.F.);
#5131=ORIENTED_EDGE('',*,*,#3803,.F.);
#5132=ORIENTED_EDGE('',*,*,#3718,.F.);
#5133=ORIENTED_EDGE('',*,*,#3802,.F.);
#5134=ORIENTED_EDGE('',*,*,#3719,.T.);
#5135=ORIENTED_EDGE('',*,*,#3803,.T.);
#5136=ORIENTED_EDGE('',*,*,#3584,.F.);
#5137=ORIENTED_EDGE('',*,*,#3393,.T.);
#5138=ORIENTED_EDGE('',*,*,#3716,.T.);
#5139=ORIENTED_EDGE('',*,*,#3391,.T.);
#5140=ORIENTED_EDGE('',*,*,#3587,.F.);
#5141=ORIENTED_EDGE('',*,*,#3498,.F.);
#5142=ORIENTED_EDGE('',*,*,#3590,.F.);
#5143=ORIENTED_EDGE('',*,*,#3804,.T.);
#5144=ORIENTED_EDGE('',*,*,#3713,.T.);
#5145=ORIENTED_EDGE('',*,*,#3506,.F.);
#5146=ORIENTED_EDGE('',*,*,#3589,.F.);
#5147=ORIENTED_EDGE('',*,*,#3805,.F.);
#5148=ORIENTED_EDGE('',*,*,#3714,.F.);
#5149=ORIENTED_EDGE('',*,*,#3804,.F.);
#5150=ORIENTED_EDGE('',*,*,#3715,.T.);
#5151=ORIENTED_EDGE('',*,*,#3805,.T.);
#5152=ORIENTED_EDGE('',*,*,#3588,.F.);
#5153=ORIENTED_EDGE('',*,*,#3389,.T.);
#5154=ORIENTED_EDGE('',*,*,#3704,.T.);
#5155=ORIENTED_EDGE('',*,*,#3387,.T.);
#5156=ORIENTED_EDGE('',*,*,#3599,.F.);
#5157=ORIENTED_EDGE('',*,*,#3494,.F.);
#5158=ORIENTED_EDGE('',*,*,#3602,.F.);
#5159=ORIENTED_EDGE('',*,*,#3806,.T.);
#5160=ORIENTED_EDGE('',*,*,#3701,.T.);
#5161=ORIENTED_EDGE('',*,*,#3492,.F.);
#5162=ORIENTED_EDGE('',*,*,#3601,.F.);
#5163=ORIENTED_EDGE('',*,*,#3807,.F.);
#5164=ORIENTED_EDGE('',*,*,#3702,.F.);
#5165=ORIENTED_EDGE('',*,*,#3806,.F.);
#5166=ORIENTED_EDGE('',*,*,#3703,.T.);
#5167=ORIENTED_EDGE('',*,*,#3807,.T.);
#5168=ORIENTED_EDGE('',*,*,#3600,.F.);
#5169=ORIENTED_EDGE('',*,*,#3385,.T.);
#5170=ORIENTED_EDGE('',*,*,#3700,.T.);
#5171=ORIENTED_EDGE('',*,*,#3808,.T.);
#5172=ORIENTED_EDGE('',*,*,#3603,.F.);
#5173=ORIENTED_EDGE('',*,*,#3490,.F.);
#5174=ORIENTED_EDGE('',*,*,#3606,.F.);
#5175=ORIENTED_EDGE('',*,*,#3381,.T.);
#5176=ORIENTED_EDGE('',*,*,#3697,.T.);
#5177=ORIENTED_EDGE('',*,*,#3488,.F.);
#5178=ORIENTED_EDGE('',*,*,#3698,.T.);
#5179=ORIENTED_EDGE('',*,*,#3383,.T.);
#5180=ORIENTED_EDGE('',*,*,#3605,.F.);
#5181=ORIENTED_EDGE('',*,*,#3809,.T.);
#5182=ORIENTED_EDGE('',*,*,#3604,.F.);
#5183=ORIENTED_EDGE('',*,*,#3808,.F.);
#5184=ORIENTED_EDGE('',*,*,#3699,.F.);
#5185=ORIENTED_EDGE('',*,*,#3809,.F.);
#5186=ORIENTED_EDGE('',*,*,#3696,.T.);
#5187=ORIENTED_EDGE('',*,*,#3810,.T.);
#5188=ORIENTED_EDGE('',*,*,#3607,.F.);
#5189=ORIENTED_EDGE('',*,*,#3486,.F.);
#5190=ORIENTED_EDGE('',*,*,#3610,.F.);
#5191=ORIENTED_EDGE('',*,*,#3377,.T.);
#5192=ORIENTED_EDGE('',*,*,#3693,.T.);
#5193=ORIENTED_EDGE('',*,*,#3484,.F.);
#5194=ORIENTED_EDGE('',*,*,#3694,.T.);
#5195=ORIENTED_EDGE('',*,*,#3379,.T.);
#5196=ORIENTED_EDGE('',*,*,#3609,.F.);
#5197=ORIENTED_EDGE('',*,*,#3811,.T.);
#5198=ORIENTED_EDGE('',*,*,#3608,.F.);
#5199=ORIENTED_EDGE('',*,*,#3810,.F.);
#5200=ORIENTED_EDGE('',*,*,#3695,.F.);
#5201=ORIENTED_EDGE('',*,*,#3811,.F.);
#5202=ORIENTED_EDGE('',*,*,#3692,.T.);
#5203=ORIENTED_EDGE('',*,*,#3812,.T.);
#5204=ORIENTED_EDGE('',*,*,#3611,.F.);
#5205=ORIENTED_EDGE('',*,*,#3482,.F.);
#5206=ORIENTED_EDGE('',*,*,#3614,.F.);
#5207=ORIENTED_EDGE('',*,*,#3373,.T.);
#5208=ORIENTED_EDGE('',*,*,#3689,.T.);
#5209=ORIENTED_EDGE('',*,*,#3476,.F.);
#5210=ORIENTED_EDGE('',*,*,#3690,.T.);
#5211=ORIENTED_EDGE('',*,*,#3375,.T.);
#5212=ORIENTED_EDGE('',*,*,#3613,.F.);
#5213=ORIENTED_EDGE('',*,*,#3813,.T.);
#5214=ORIENTED_EDGE('',*,*,#3612,.F.);
#5215=ORIENTED_EDGE('',*,*,#3812,.F.);
#5216=ORIENTED_EDGE('',*,*,#3691,.F.);
#5217=ORIENTED_EDGE('',*,*,#3813,.F.);
#5218=ORIENTED_EDGE('',*,*,#3684,.T.);
#5219=ORIENTED_EDGE('',*,*,#3814,.T.);
#5220=ORIENTED_EDGE('',*,*,#3619,.F.);
#5221=ORIENTED_EDGE('',*,*,#3480,.F.);
#5222=ORIENTED_EDGE('',*,*,#3622,.F.);
#5223=ORIENTED_EDGE('',*,*,#3369,.T.);
#5224=ORIENTED_EDGE('',*,*,#3681,.T.);
#5225=ORIENTED_EDGE('',*,*,#3472,.F.);
#5226=ORIENTED_EDGE('',*,*,#3682,.T.);
#5227=ORIENTED_EDGE('',*,*,#3371,.T.);
#5228=ORIENTED_EDGE('',*,*,#3621,.F.);
#5229=ORIENTED_EDGE('',*,*,#3815,.T.);
#5230=ORIENTED_EDGE('',*,*,#3620,.F.);
#5231=ORIENTED_EDGE('',*,*,#3814,.F.);
#5232=ORIENTED_EDGE('',*,*,#3683,.F.);
#5233=ORIENTED_EDGE('',*,*,#3815,.F.);
#5234=ORIENTED_EDGE('',*,*,#3688,.T.);
#5235=ORIENTED_EDGE('',*,*,#3816,.T.);
#5236=ORIENTED_EDGE('',*,*,#3615,.F.);
#5237=ORIENTED_EDGE('',*,*,#3474,.F.);
#5238=ORIENTED_EDGE('',*,*,#3618,.F.);
#5239=ORIENTED_EDGE('',*,*,#3365,.T.);
#5240=ORIENTED_EDGE('',*,*,#3685,.T.);
#5241=ORIENTED_EDGE('',*,*,#3478,.F.);
#5242=ORIENTED_EDGE('',*,*,#3686,.T.);
#5243=ORIENTED_EDGE('',*,*,#3367,.T.);
#5244=ORIENTED_EDGE('',*,*,#3617,.F.);
#5245=ORIENTED_EDGE('',*,*,#3817,.T.);
#5246=ORIENTED_EDGE('',*,*,#3616,.F.);
#5247=ORIENTED_EDGE('',*,*,#3816,.F.);
#5248=ORIENTED_EDGE('',*,*,#3687,.F.);
#5249=ORIENTED_EDGE('',*,*,#3817,.F.);
#5250=ORIENTED_EDGE('',*,*,#3680,.T.);
#5251=ORIENTED_EDGE('',*,*,#3818,.T.);
#5252=ORIENTED_EDGE('',*,*,#3623,.F.);
#5253=ORIENTED_EDGE('',*,*,#3470,.F.);
#5254=ORIENTED_EDGE('',*,*,#3678,.T.);
#5255=ORIENTED_EDGE('',*,*,#3360,.T.);
#5256=ORIENTED_EDGE('',*,*,#3625,.F.);
#5257=ORIENTED_EDGE('',*,*,#3819,.T.);
#5258=ORIENTED_EDGE('',*,*,#3624,.F.);
#5259=ORIENTED_EDGE('',*,*,#3818,.F.);
#5260=ORIENTED_EDGE('',*,*,#3679,.F.);
#5261=ORIENTED_EDGE('',*,*,#3819,.F.);
#5262=ORIENTED_EDGE('',*,*,#3677,.T.);
#5263=ORIENTED_EDGE('',*,*,#3820,.T.);
#5264=ORIENTED_EDGE('',*,*,#3626,.F.);
#5265=ORIENTED_EDGE('',*,*,#3467,.F.);
#5266=ORIENTED_EDGE('',*,*,#3675,.T.);
#5267=ORIENTED_EDGE('',*,*,#3353,.T.);
#5268=ORIENTED_EDGE('',*,*,#3628,.F.);
#5269=ORIENTED_EDGE('',*,*,#3821,.T.);
#5270=ORIENTED_EDGE('',*,*,#3627,.F.);
#5271=ORIENTED_EDGE('',*,*,#3820,.F.);
#5272=ORIENTED_EDGE('',*,*,#3676,.F.);
#5273=ORIENTED_EDGE('',*,*,#3821,.F.);
#5274=ORIENTED_EDGE('',*,*,#3582,.F.);
#5275=ORIENTED_EDGE('',*,*,#3822,.T.);
#5276=ORIENTED_EDGE('',*,*,#3721,.T.);
#5277=ORIENTED_EDGE('',*,*,#3502,.F.);
#5278=ORIENTED_EDGE('',*,*,#3581,.F.);
#5279=ORIENTED_EDGE('',*,*,#3823,.F.);
#5280=ORIENTED_EDGE('',*,*,#3722,.F.);
#5281=ORIENTED_EDGE('',*,*,#3822,.F.);
#5282=ORIENTED_EDGE('',*,*,#3723,.T.);
#5283=ORIENTED_EDGE('',*,*,#3823,.T.);
#5284=ORIENTED_EDGE('',*,*,#3580,.F.);
#5285=ORIENTED_EDGE('',*,*,#3344,.T.);
#5286=ORIENTED_EDGE('',*,*,#3579,.F.);
#5287=ORIENTED_EDGE('',*,*,#3824,.T.);
#5288=ORIENTED_EDGE('',*,*,#3724,.T.);
#5289=ORIENTED_EDGE('',*,*,#3464,.F.);
#5290=ORIENTED_EDGE('',*,*,#3578,.F.);
#5291=ORIENTED_EDGE('',*,*,#3825,.F.);
#5292=ORIENTED_EDGE('',*,*,#3725,.F.);
#5293=ORIENTED_EDGE('',*,*,#3824,.F.);
#5294=ORIENTED_EDGE('',*,*,#3726,.T.);
#5295=ORIENTED_EDGE('',*,*,#3825,.T.);
#5296=ORIENTED_EDGE('',*,*,#3577,.F.);
#5297=ORIENTED_EDGE('',*,*,#3337,.T.);
#5298=ORIENTED_EDGE('',*,*,#3731,.T.);
#5299=ORIENTED_EDGE('',*,*,#3826,.T.);
#5300=ORIENTED_EDGE('',*,*,#3572,.F.);
#5301=ORIENTED_EDGE('',*,*,#3459,.F.);
#5302=ORIENTED_EDGE('',*,*,#3576,.F.);
#5303=ORIENTED_EDGE('',*,*,#3827,.T.);
#5304=ORIENTED_EDGE('',*,*,#3727,.T.);
#5305=ORIENTED_EDGE('',*,*,#3461,.F.);
#5306=ORIENTED_EDGE('',*,*,#3575,.F.);
#5307=ORIENTED_EDGE('',*,*,#3828,.F.);
#5308=ORIENTED_EDGE('',*,*,#3728,.F.);
#5309=ORIENTED_EDGE('',*,*,#3827,.F.);
#5310=ORIENTED_EDGE('',*,*,#3729,.T.);
#5311=ORIENTED_EDGE('',*,*,#3828,.T.);
#5312=ORIENTED_EDGE('',*,*,#3574,.F.);
#5313=ORIENTED_EDGE('',*,*,#3829,.T.);
#5314=ORIENTED_EDGE('',*,*,#3573,.F.);
#5315=ORIENTED_EDGE('',*,*,#3826,.F.);
#5316=ORIENTED_EDGE('',*,*,#3730,.F.);
#5317=ORIENTED_EDGE('',*,*,#3829,.F.);
#5318=ORIENTED_EDGE('',*,*,#3736,.T.);
#5319=ORIENTED_EDGE('',*,*,#3830,.T.);
#5320=ORIENTED_EDGE('',*,*,#3567,.F.);
#5321=ORIENTED_EDGE('',*,*,#3455,.F.);
#5322=ORIENTED_EDGE('',*,*,#3571,.F.);
#5323=ORIENTED_EDGE('',*,*,#3831,.T.);
#5324=ORIENTED_EDGE('',*,*,#3732,.T.);
#5325=ORIENTED_EDGE('',*,*,#3457,.F.);
#5326=ORIENTED_EDGE('',*,*,#3570,.F.);
#5327=ORIENTED_EDGE('',*,*,#3832,.F.);
#5328=ORIENTED_EDGE('',*,*,#3733,.F.);
#5329=ORIENTED_EDGE('',*,*,#3831,.F.);
#5330=ORIENTED_EDGE('',*,*,#3734,.T.);
#5331=ORIENTED_EDGE('',*,*,#3832,.T.);
#5332=ORIENTED_EDGE('',*,*,#3569,.F.);
#5333=ORIENTED_EDGE('',*,*,#3833,.T.);
#5334=ORIENTED_EDGE('',*,*,#3568,.F.);
#5335=ORIENTED_EDGE('',*,*,#3830,.F.);
#5336=ORIENTED_EDGE('',*,*,#3735,.F.);
#5337=ORIENTED_EDGE('',*,*,#3833,.F.);
#5338=ORIENTED_EDGE('',*,*,#3751,.T.);
#5339=ORIENTED_EDGE('',*,*,#3834,.T.);
#5340=ORIENTED_EDGE('',*,*,#3552,.F.);
#5341=ORIENTED_EDGE('',*,*,#3451,.F.);
#5342=ORIENTED_EDGE('',*,*,#3556,.F.);
#5343=ORIENTED_EDGE('',*,*,#3835,.T.);
#5344=ORIENTED_EDGE('',*,*,#3747,.T.);
#5345=ORIENTED_EDGE('',*,*,#3443,.F.);
#5346=ORIENTED_EDGE('',*,*,#3555,.F.);
#5347=ORIENTED_EDGE('',*,*,#3836,.F.);
#5348=ORIENTED_EDGE('',*,*,#3748,.F.);
#5349=ORIENTED_EDGE('',*,*,#3835,.F.);
#5350=ORIENTED_EDGE('',*,*,#3749,.T.);
#5351=ORIENTED_EDGE('',*,*,#3836,.T.);
#5352=ORIENTED_EDGE('',*,*,#3554,.F.);
#5353=ORIENTED_EDGE('',*,*,#3837,.T.);
#5354=ORIENTED_EDGE('',*,*,#3553,.F.);
#5355=ORIENTED_EDGE('',*,*,#3834,.F.);
#5356=ORIENTED_EDGE('',*,*,#3750,.F.);
#5357=ORIENTED_EDGE('',*,*,#3837,.F.);
#5358=ORIENTED_EDGE('',*,*,#3756,.T.);
#5359=ORIENTED_EDGE('',*,*,#3838,.T.);
#5360=ORIENTED_EDGE('',*,*,#3547,.F.);
#5361=ORIENTED_EDGE('',*,*,#3447,.F.);
#5362=ORIENTED_EDGE('',*,*,#3551,.F.);
#5363=ORIENTED_EDGE('',*,*,#3839,.T.);
#5364=ORIENTED_EDGE('',*,*,#3752,.T.);
#5365=ORIENTED_EDGE('',*,*,#3449,.F.);
#5366=ORIENTED_EDGE('',*,*,#3550,.F.);
#5367=ORIENTED_EDGE('',*,*,#3840,.F.);
#5368=ORIENTED_EDGE('',*,*,#3753,.F.);
#5369=ORIENTED_EDGE('',*,*,#3839,.F.);
#5370=ORIENTED_EDGE('',*,*,#3754,.T.);
#5371=ORIENTED_EDGE('',*,*,#3840,.T.);
#5372=ORIENTED_EDGE('',*,*,#3549,.F.);
#5373=ORIENTED_EDGE('',*,*,#3841,.T.);
#5374=ORIENTED_EDGE('',*,*,#3548,.F.);
#5375=ORIENTED_EDGE('',*,*,#3838,.F.);
#5376=ORIENTED_EDGE('',*,*,#3755,.F.);
#5377=ORIENTED_EDGE('',*,*,#3841,.F.);
#5378=ORIENTED_EDGE('',*,*,#3746,.T.);
#5379=ORIENTED_EDGE('',*,*,#3842,.T.);
#5380=ORIENTED_EDGE('',*,*,#3557,.F.);
#5381=ORIENTED_EDGE('',*,*,#3441,.F.);
#5382=ORIENTED_EDGE('',*,*,#3561,.F.);
#5383=ORIENTED_EDGE('',*,*,#3843,.T.);
#5384=ORIENTED_EDGE('',*,*,#3742,.T.);
#5385=ORIENTED_EDGE('',*,*,#3439,.F.);
#5386=ORIENTED_EDGE('',*,*,#3560,.F.);
#5387=ORIENTED_EDGE('',*,*,#3844,.F.);
#5388=ORIENTED_EDGE('',*,*,#3743,.F.);
#5389=ORIENTED_EDGE('',*,*,#3843,.F.);
#5390=ORIENTED_EDGE('',*,*,#3744,.T.);
#5391=ORIENTED_EDGE('',*,*,#3844,.T.);
#5392=ORIENTED_EDGE('',*,*,#3559,.F.);
#5393=ORIENTED_EDGE('',*,*,#3845,.T.);
#5394=ORIENTED_EDGE('',*,*,#3558,.F.);
#5395=ORIENTED_EDGE('',*,*,#3842,.F.);
#5396=ORIENTED_EDGE('',*,*,#3745,.F.);
#5397=ORIENTED_EDGE('',*,*,#3845,.F.);
#5398=ORIENTED_EDGE('',*,*,#3741,.T.);
#5399=ORIENTED_EDGE('',*,*,#3846,.T.);
#5400=ORIENTED_EDGE('',*,*,#3562,.F.);
#5401=ORIENTED_EDGE('',*,*,#3437,.F.);
#5402=ORIENTED_EDGE('',*,*,#3566,.F.);
#5403=ORIENTED_EDGE('',*,*,#3847,.T.);
#5404=ORIENTED_EDGE('',*,*,#3737,.T.);
#5405=ORIENTED_EDGE('',*,*,#3453,.F.);
#5406=ORIENTED_EDGE('',*,*,#3565,.F.);
#5407=ORIENTED_EDGE('',*,*,#3848,.F.);
#5408=ORIENTED_EDGE('',*,*,#3738,.F.);
#5409=ORIENTED_EDGE('',*,*,#3847,.F.);
#5410=ORIENTED_EDGE('',*,*,#3739,.T.);
#5411=ORIENTED_EDGE('',*,*,#3848,.T.);
#5412=ORIENTED_EDGE('',*,*,#3564,.F.);
#5413=ORIENTED_EDGE('',*,*,#3849,.T.);
#5414=ORIENTED_EDGE('',*,*,#3563,.F.);
#5415=ORIENTED_EDGE('',*,*,#3846,.F.);
#5416=ORIENTED_EDGE('',*,*,#3740,.F.);
#5417=ORIENTED_EDGE('',*,*,#3849,.F.);
#5418=ORIENTED_EDGE('',*,*,#3761,.T.);
#5419=ORIENTED_EDGE('',*,*,#3850,.T.);
#5420=ORIENTED_EDGE('',*,*,#3542,.F.);
#5421=ORIENTED_EDGE('',*,*,#3435,.F.);
#5422=ORIENTED_EDGE('',*,*,#3546,.F.);
#5423=ORIENTED_EDGE('',*,*,#3851,.T.);
#5424=ORIENTED_EDGE('',*,*,#3757,.T.);
#5425=ORIENTED_EDGE('',*,*,#3445,.F.);
#5426=ORIENTED_EDGE('',*,*,#3545,.F.);
#5427=ORIENTED_EDGE('',*,*,#3852,.F.);
#5428=ORIENTED_EDGE('',*,*,#3758,.F.);
#5429=ORIENTED_EDGE('',*,*,#3851,.F.);
#5430=ORIENTED_EDGE('',*,*,#3759,.T.);
#5431=ORIENTED_EDGE('',*,*,#3852,.T.);
#5432=ORIENTED_EDGE('',*,*,#3544,.F.);
#5433=ORIENTED_EDGE('',*,*,#3853,.T.);
#5434=ORIENTED_EDGE('',*,*,#3543,.F.);
#5435=ORIENTED_EDGE('',*,*,#3850,.F.);
#5436=ORIENTED_EDGE('',*,*,#3760,.F.);
#5437=ORIENTED_EDGE('',*,*,#3853,.F.);
#5438=ORIENTED_EDGE('',*,*,#3766,.T.);
#5439=ORIENTED_EDGE('',*,*,#3854,.T.);
#5440=ORIENTED_EDGE('',*,*,#3537,.F.);
#5441=ORIENTED_EDGE('',*,*,#3405,.F.);
#5442=ORIENTED_EDGE('',*,*,#3541,.F.);
#5443=ORIENTED_EDGE('',*,*,#3855,.T.);
#5444=ORIENTED_EDGE('',*,*,#3762,.T.);
#5445=ORIENTED_EDGE('',*,*,#3433,.F.);
#5446=ORIENTED_EDGE('',*,*,#3540,.F.);
#5447=ORIENTED_EDGE('',*,*,#3856,.F.);
#5448=ORIENTED_EDGE('',*,*,#3763,.F.);
#5449=ORIENTED_EDGE('',*,*,#3855,.F.);
#5450=ORIENTED_EDGE('',*,*,#3764,.T.);
#5451=ORIENTED_EDGE('',*,*,#3856,.T.);
#5452=ORIENTED_EDGE('',*,*,#3539,.F.);
#5453=ORIENTED_EDGE('',*,*,#3857,.T.);
#5454=ORIENTED_EDGE('',*,*,#3538,.F.);
#5455=ORIENTED_EDGE('',*,*,#3854,.F.);
#5456=ORIENTED_EDGE('',*,*,#3765,.F.);
#5457=ORIENTED_EDGE('',*,*,#3857,.F.);
#5458=ORIENTED_EDGE('',*,*,#3771,.T.);
#5459=ORIENTED_EDGE('',*,*,#3858,.T.);
#5460=ORIENTED_EDGE('',*,*,#3532,.F.);
#5461=ORIENTED_EDGE('',*,*,#3431,.F.);
#5462=ORIENTED_EDGE('',*,*,#3536,.F.);
#5463=ORIENTED_EDGE('',*,*,#3859,.T.);
#5464=ORIENTED_EDGE('',*,*,#3767,.T.);
#5465=ORIENTED_EDGE('',*,*,#3407,.F.);
#5466=ORIENTED_EDGE('',*,*,#3535,.F.);
#5467=ORIENTED_EDGE('',*,*,#3860,.F.);
#5468=ORIENTED_EDGE('',*,*,#3768,.F.);
#5469=ORIENTED_EDGE('',*,*,#3859,.F.);
#5470=ORIENTED_EDGE('',*,*,#3769,.T.);
#5471=ORIENTED_EDGE('',*,*,#3860,.T.);
#5472=ORIENTED_EDGE('',*,*,#3534,.F.);
#5473=ORIENTED_EDGE('',*,*,#3861,.T.);
#5474=ORIENTED_EDGE('',*,*,#3533,.F.);
#5475=ORIENTED_EDGE('',*,*,#3858,.F.);
#5476=ORIENTED_EDGE('',*,*,#3770,.F.);
#5477=ORIENTED_EDGE('',*,*,#3861,.F.);
#5478=ORIENTED_EDGE('',*,*,#3776,.T.);
#5479=ORIENTED_EDGE('',*,*,#3862,.T.);
#5480=ORIENTED_EDGE('',*,*,#3527,.F.);
#5481=ORIENTED_EDGE('',*,*,#3427,.F.);
#5482=ORIENTED_EDGE('',*,*,#3531,.F.);
#5483=ORIENTED_EDGE('',*,*,#3863,.T.);
#5484=ORIENTED_EDGE('',*,*,#3772,.T.);
#5485=ORIENTED_EDGE('',*,*,#3429,.F.);
#5486=ORIENTED_EDGE('',*,*,#3530,.F.);
#5487=ORIENTED_EDGE('',*,*,#3864,.F.);
#5488=ORIENTED_EDGE('',*,*,#3773,.F.);
#5489=ORIENTED_EDGE('',*,*,#3863,.F.);
#5490=ORIENTED_EDGE('',*,*,#3774,.T.);
#5491=ORIENTED_EDGE('',*,*,#3864,.T.);
#5492=ORIENTED_EDGE('',*,*,#3529,.F.);
#5493=ORIENTED_EDGE('',*,*,#3865,.T.);
#5494=ORIENTED_EDGE('',*,*,#3528,.F.);
#5495=ORIENTED_EDGE('',*,*,#3862,.F.);
#5496=ORIENTED_EDGE('',*,*,#3775,.F.);
#5497=ORIENTED_EDGE('',*,*,#3865,.F.);
#5498=ORIENTED_EDGE('',*,*,#3663,.T.);
#5499=ORIENTED_EDGE('',*,*,#3866,.T.);
#5500=ORIENTED_EDGE('',*,*,#3640,.F.);
#5501=ORIENTED_EDGE('',*,*,#3421,.F.);
#5502=ORIENTED_EDGE('',*,*,#3644,.F.);
#5503=ORIENTED_EDGE('',*,*,#3867,.T.);
#5504=ORIENTED_EDGE('',*,*,#3659,.T.);
#5505=ORIENTED_EDGE('',*,*,#3419,.F.);
#5506=ORIENTED_EDGE('',*,*,#3643,.F.);
#5507=ORIENTED_EDGE('',*,*,#3868,.F.);
#5508=ORIENTED_EDGE('',*,*,#3660,.F.);
#5509=ORIENTED_EDGE('',*,*,#3867,.F.);
#5510=ORIENTED_EDGE('',*,*,#3661,.T.);
#5511=ORIENTED_EDGE('',*,*,#3868,.T.);
#5512=ORIENTED_EDGE('',*,*,#3642,.F.);
#5513=ORIENTED_EDGE('',*,*,#3869,.T.);
#5514=ORIENTED_EDGE('',*,*,#3641,.F.);
#5515=ORIENTED_EDGE('',*,*,#3866,.F.);
#5516=ORIENTED_EDGE('',*,*,#3662,.F.);
#5517=ORIENTED_EDGE('',*,*,#3869,.F.);
#5518=ORIENTED_EDGE('',*,*,#3658,.T.);
#5519=ORIENTED_EDGE('',*,*,#3870,.T.);
#5520=ORIENTED_EDGE('',*,*,#3645,.F.);
#5521=ORIENTED_EDGE('',*,*,#3417,.F.);
#5522=ORIENTED_EDGE('',*,*,#3649,.F.);
#5523=ORIENTED_EDGE('',*,*,#3871,.T.);
#5524=ORIENTED_EDGE('',*,*,#3654,.T.);
#5525=ORIENTED_EDGE('',*,*,#3411,.F.);
#5526=ORIENTED_EDGE('',*,*,#3648,.F.);
#5527=ORIENTED_EDGE('',*,*,#3872,.F.);
#5528=ORIENTED_EDGE('',*,*,#3655,.F.);
#5529=ORIENTED_EDGE('',*,*,#3871,.F.);
#5530=ORIENTED_EDGE('',*,*,#3656,.T.);
#5531=ORIENTED_EDGE('',*,*,#3872,.T.);
#5532=ORIENTED_EDGE('',*,*,#3647,.F.);
#5533=ORIENTED_EDGE('',*,*,#3873,.T.);
#5534=ORIENTED_EDGE('',*,*,#3646,.F.);
#5535=ORIENTED_EDGE('',*,*,#3870,.F.);
#5536=ORIENTED_EDGE('',*,*,#3657,.F.);
#5537=ORIENTED_EDGE('',*,*,#3873,.F.);
#5538=ORIENTED_EDGE('',*,*,#3781,.T.);
#5539=ORIENTED_EDGE('',*,*,#3874,.T.);
#5540=ORIENTED_EDGE('',*,*,#3522,.F.);
#5541=ORIENTED_EDGE('',*,*,#3415,.F.);
#5542=ORIENTED_EDGE('',*,*,#3526,.F.);
#5543=ORIENTED_EDGE('',*,*,#3875,.T.);
#5544=ORIENTED_EDGE('',*,*,#3777,.T.);
#5545=ORIENTED_EDGE('',*,*,#3425,.F.);
#5546=ORIENTED_EDGE('',*,*,#3525,.F.);
#5547=ORIENTED_EDGE('',*,*,#3876,.F.);
#5548=ORIENTED_EDGE('',*,*,#3778,.F.);
#5549=ORIENTED_EDGE('',*,*,#3875,.F.);
#5550=ORIENTED_EDGE('',*,*,#3779,.T.);
#5551=ORIENTED_EDGE('',*,*,#3876,.T.);
#5552=ORIENTED_EDGE('',*,*,#3524,.F.);
#5553=ORIENTED_EDGE('',*,*,#3877,.T.);
#5554=ORIENTED_EDGE('',*,*,#3523,.F.);
#5555=ORIENTED_EDGE('',*,*,#3874,.F.);
#5556=ORIENTED_EDGE('',*,*,#3780,.F.);
#5557=ORIENTED_EDGE('',*,*,#3877,.F.);
#5558=ORIENTED_EDGE('',*,*,#3653,.T.);
#5559=ORIENTED_EDGE('',*,*,#3878,.T.);
#5560=ORIENTED_EDGE('',*,*,#3517,.F.);
#5561=ORIENTED_EDGE('',*,*,#3409,.F.);
#5562=ORIENTED_EDGE('',*,*,#3521,.F.);
#5563=ORIENTED_EDGE('',*,*,#3879,.T.);
#5564=ORIENTED_EDGE('',*,*,#3782,.T.);
#5565=ORIENTED_EDGE('',*,*,#3413,.F.);
#5566=ORIENTED_EDGE('',*,*,#3520,.F.);
#5567=ORIENTED_EDGE('',*,*,#3880,.F.);
#5568=ORIENTED_EDGE('',*,*,#3783,.F.);
#5569=ORIENTED_EDGE('',*,*,#3879,.F.);
#5570=ORIENTED_EDGE('',*,*,#3784,.T.);
#5571=ORIENTED_EDGE('',*,*,#3880,.T.);
#5572=ORIENTED_EDGE('',*,*,#3519,.F.);
#5573=ORIENTED_EDGE('',*,*,#3881,.T.);
#5574=ORIENTED_EDGE('',*,*,#3518,.F.);
#5575=ORIENTED_EDGE('',*,*,#3878,.F.);
#5576=ORIENTED_EDGE('',*,*,#3785,.F.);
#5577=ORIENTED_EDGE('',*,*,#3881,.F.);
#5578=ORIENTED_EDGE('',*,*,#3786,.T.);
#5579=ORIENTED_EDGE('',*,*,#3333,.F.);
#5580=ORIENTED_EDGE('',*,*,#3650,.F.);
#5581=ORIENTED_EDGE('',*,*,#3882,.T.);
#5582=ORIENTED_EDGE('',*,*,#3787,.T.);
#5583=ORIENTED_EDGE('',*,*,#3882,.F.);
#5584=ORIENTED_EDGE('',*,*,#3652,.F.);
#5585=ORIENTED_EDGE('',*,*,#3883,.T.);
#5586=ORIENTED_EDGE('',*,*,#3788,.T.);
#5587=ORIENTED_EDGE('',*,*,#3883,.F.);
#5588=ORIENTED_EDGE('',*,*,#3651,.F.);
#5589=ORIENTED_EDGE('',*,*,#3335,.T.);
#6079=CYLINDRICAL_SURFACE('',#6900,3.);
#6080=CYLINDRICAL_SURFACE('',#6903,0.27);
#6081=CYLINDRICAL_SURFACE('',#6906,3.68751484013274);
#6082=CYLINDRICAL_SURFACE('',#6909,0.27);
#6083=CYLINDRICAL_SURFACE('',#6912,3.68751484013274);
#6084=CYLINDRICAL_SURFACE('',#6915,0.27);
#6085=CYLINDRICAL_SURFACE('',#6918,3.68751484013274);
#6086=CYLINDRICAL_SURFACE('',#6921,0.269999999999999);
#6087=CYLINDRICAL_SURFACE('',#6924,3.68751484013274);
#6088=CYLINDRICAL_SURFACE('',#6927,0.269999999999999);
#6089=CYLINDRICAL_SURFACE('',#6930,0.269999999999999);
#6090=CYLINDRICAL_SURFACE('',#6933,0.269999999999999);
#6091=CYLINDRICAL_SURFACE('',#6936,0.269999999999999);
#6092=CYLINDRICAL_SURFACE('',#6939,0.269999999999999);
#6093=CYLINDRICAL_SURFACE('',#6942,0.269999999999999);
#6094=CYLINDRICAL_SURFACE('',#6945,0.269999999999999);
#6095=CYLINDRICAL_SURFACE('',#6948,0.269999999999999);
#6096=CYLINDRICAL_SURFACE('',#6951,0.269999999999999);
#6097=CYLINDRICAL_SURFACE('',#6954,0.269999999999999);
#6098=CYLINDRICAL_SURFACE('',#6957,14.4);
#6099=CYLINDRICAL_SURFACE('',#6960,14.4);
#6100=CYLINDRICAL_SURFACE('',#6963,14.4);
#6101=CYLINDRICAL_SURFACE('',#6966,14.4);
#6102=CYLINDRICAL_SURFACE('',#6969,14.4);
#6103=CYLINDRICAL_SURFACE('',#6972,14.4);
#6104=CYLINDRICAL_SURFACE('',#6975,14.4);
#6105=CYLINDRICAL_SURFACE('',#6978,14.4);
#6106=CYLINDRICAL_SURFACE('',#6981,14.4);
#6107=CYLINDRICAL_SURFACE('',#6984,14.4);
#6108=CYLINDRICAL_SURFACE('',#6987,14.4);
#6109=CYLINDRICAL_SURFACE('',#6990,14.4);
#6110=CYLINDRICAL_SURFACE('',#6993,14.4);
#6111=CYLINDRICAL_SURFACE('',#6996,14.4);
#6112=CYLINDRICAL_SURFACE('',#6999,14.4);
#6113=CYLINDRICAL_SURFACE('',#7002,14.4);
#6114=CYLINDRICAL_SURFACE('',#7005,14.4);
#6115=CYLINDRICAL_SURFACE('',#7008,14.4);
#6116=CYLINDRICAL_SURFACE('',#7011,14.4);
#6117=CYLINDRICAL_SURFACE('',#7014,14.4);
#6118=CYLINDRICAL_SURFACE('',#7017,14.4);
#6119=CYLINDRICAL_SURFACE('',#7020,14.4);
#6120=CYLINDRICAL_SURFACE('',#7023,14.4);
#6121=CYLINDRICAL_SURFACE('',#7026,14.4);
#6122=CYLINDRICAL_SURFACE('',#7029,14.4);
#6123=CYLINDRICAL_SURFACE('',#7032,14.4);
#6124=CYLINDRICAL_SURFACE('',#7035,14.4);
#6125=CYLINDRICAL_SURFACE('',#7038,14.4);
#6126=CYLINDRICAL_SURFACE('',#7041,14.4);
#6127=CYLINDRICAL_SURFACE('',#7312,14.4);
#6128=CYLINDRICAL_SURFACE('',#7313,3.68751484013274);
#6129=CYLINDRICAL_SURFACE('',#7314,3.68751484013274);
#6130=CYLINDRICAL_SURFACE('',#7315,12.375);
#6131=CYLINDRICAL_SURFACE('',#7316,0.27);
#6132=CYLINDRICAL_SURFACE('',#7317,0.27);
#6133=CYLINDRICAL_SURFACE('',#7318,3.68751484013274);
#6134=CYLINDRICAL_SURFACE('',#7319,3.68751484013274);
#6135=CYLINDRICAL_SURFACE('',#7320,0.27);
#6136=CYLINDRICAL_SURFACE('',#7321,12.375);
#6137=CYLINDRICAL_SURFACE('',#7322,0.27);
#6138=CYLINDRICAL_SURFACE('',#7323,3.68751484013274);
#6139=CYLINDRICAL_SURFACE('',#7324,3.68751484013274);
#6140=CYLINDRICAL_SURFACE('',#7325,0.269999999999999);
#6141=CYLINDRICAL_SURFACE('',#7326,12.375);
#6142=CYLINDRICAL_SURFACE('',#7327,3.68751484013274);
#6143=CYLINDRICAL_SURFACE('',#7328,3.68751484013274);
#6144=CYLINDRICAL_SURFACE('',#7329,0.269999999999999);
#6145=CYLINDRICAL_SURFACE('',#7330,12.375);
#6146=CYLINDRICAL_SURFACE('',#7331,3.68751484013274);
#6147=CYLINDRICAL_SURFACE('',#7332,3.68751484013274);
#6148=CYLINDRICAL_SURFACE('',#7333,0.269999999999999);
#6149=CYLINDRICAL_SURFACE('',#7334,12.375);
#6150=CYLINDRICAL_SURFACE('',#7335,3.68751484013274);
#6151=CYLINDRICAL_SURFACE('',#7336,3.68751484013274);
#6152=CYLINDRICAL_SURFACE('',#7337,0.269999999999999);
#6153=CYLINDRICAL_SURFACE('',#7338,12.375);
#6154=CYLINDRICAL_SURFACE('',#7339,3.68751484013274);
#6155=CYLINDRICAL_SURFACE('',#7340,3.68751484013274);
#6156=CYLINDRICAL_SURFACE('',#7341,0.269999999999999);
#6157=CYLINDRICAL_SURFACE('',#7342,12.375);
#6158=CYLINDRICAL_SURFACE('',#7343,3.68751484013274);
#6159=CYLINDRICAL_SURFACE('',#7344,3.68751484013274);
#6160=CYLINDRICAL_SURFACE('',#7345,12.375);
#6161=CYLINDRICAL_SURFACE('',#7346,0.269999999999999);
#6162=CYLINDRICAL_SURFACE('',#7347,3.68751484013274);
#6163=CYLINDRICAL_SURFACE('',#7348,3.68751484013274);
#6164=CYLINDRICAL_SURFACE('',#7349,12.375);
#6165=CYLINDRICAL_SURFACE('',#7350,0.269999999999999);
#6166=CYLINDRICAL_SURFACE('',#7351,3.68751484013274);
#6167=CYLINDRICAL_SURFACE('',#7352,3.68751484013274);
#6168=CYLINDRICAL_SURFACE('',#7353,12.375);
#6169=CYLINDRICAL_SURFACE('',#7354,0.269999999999999);
#6170=CYLINDRICAL_SURFACE('',#7355,3.68751484013274);
#6171=CYLINDRICAL_SURFACE('',#7356,3.68751484013274);
#6172=CYLINDRICAL_SURFACE('',#7357,12.375);
#6173=CYLINDRICAL_SURFACE('',#7358,0.27);
#6174=CYLINDRICAL_SURFACE('',#7359,3.68751484013274);
#6175=CYLINDRICAL_SURFACE('',#7360,3.68751484013274);
#6176=CYLINDRICAL_SURFACE('',#7361,12.375);
#6177=CYLINDRICAL_SURFACE('',#7362,0.269999999999999);
#6178=CYLINDRICAL_SURFACE('',#7363,3.68751484013274);
#6179=CYLINDRICAL_SURFACE('',#7364,12.375);
#6180=CYLINDRICAL_SURFACE('',#7365,0.269999999999999);
#6181=CYLINDRICAL_SURFACE('',#7366,3.68751484013274);
#6182=CYLINDRICAL_SURFACE('',#7367,12.375);
#6183=CYLINDRICAL_SURFACE('',#7368,0.27);
#6184=CYLINDRICAL_SURFACE('',#7369,3.68751484013274);
#6185=CYLINDRICAL_SURFACE('',#7370,0.269999999999999);
#6186=CYLINDRICAL_SURFACE('',#7371,12.375);
#6187=CYLINDRICAL_SURFACE('',#7372,3.68751484013274);
#6188=CYLINDRICAL_SURFACE('',#7373,0.27);
#6189=CYLINDRICAL_SURFACE('',#7374,12.375);
#6190=CYLINDRICAL_SURFACE('',#7375,3.68751484013274);
#6191=CYLINDRICAL_SURFACE('',#7376,3.68751484013274);
#6192=CYLINDRICAL_SURFACE('',#7377,0.27);
#6193=CYLINDRICAL_SURFACE('',#7378,12.375);
#6194=CYLINDRICAL_SURFACE('',#7379,0.27);
#6195=CYLINDRICAL_SURFACE('',#7380,3.68751484013274);
#6196=CYLINDRICAL_SURFACE('',#7381,3.68751484013274);
#6197=CYLINDRICAL_SURFACE('',#7382,0.27);
#6198=CYLINDRICAL_SURFACE('',#7383,12.375);
#6199=CYLINDRICAL_SURFACE('',#7384,0.27);
#6200=CYLINDRICAL_SURFACE('',#7385,3.68751484013274);
#6201=CYLINDRICAL_SURFACE('',#7386,3.68751484013274);
#6202=CYLINDRICAL_SURFACE('',#7387,0.269999999999999);
#6203=CYLINDRICAL_SURFACE('',#7388,12.375);
#6204=CYLINDRICAL_SURFACE('',#7389,0.269999999999999);
#6205=CYLINDRICAL_SURFACE('',#7390,3.68751484013274);
#6206=CYLINDRICAL_SURFACE('',#7391,3.68751484013274);
#6207=CYLINDRICAL_SURFACE('',#7392,0.269999999999999);
#6208=CYLINDRICAL_SURFACE('',#7393,12.375);
#6209=CYLINDRICAL_SURFACE('',#7394,0.269999999999999);
#6210=CYLINDRICAL_SURFACE('',#7395,3.68751484013274);
#6211=CYLINDRICAL_SURFACE('',#7396,3.68751484013274);
#6212=CYLINDRICAL_SURFACE('',#7397,0.269999999999999);
#6213=CYLINDRICAL_SURFACE('',#7398,12.375);
#6214=CYLINDRICAL_SURFACE('',#7399,0.269999999999999);
#6215=CYLINDRICAL_SURFACE('',#7400,3.68751484013274);
#6216=CYLINDRICAL_SURFACE('',#7401,3.68751484013274);
#6217=CYLINDRICAL_SURFACE('',#7402,0.27);
#6218=CYLINDRICAL_SURFACE('',#7403,12.375);
#6219=CYLINDRICAL_SURFACE('',#7404,0.269999999999999);
#6220=CYLINDRICAL_SURFACE('',#7405,3.68751484013274);
#6221=CYLINDRICAL_SURFACE('',#7406,3.68751484013274);
#6222=CYLINDRICAL_SURFACE('',#7407,0.269999999999999);
#6223=CYLINDRICAL_SURFACE('',#7408,12.375);
#6224=CYLINDRICAL_SURFACE('',#7409,0.269999999999999);
#6225=CYLINDRICAL_SURFACE('',#7410,3.68751484013274);
#6226=CYLINDRICAL_SURFACE('',#7411,3.68751484013274);
#6227=CYLINDRICAL_SURFACE('',#7412,0.269999999999999);
#6228=CYLINDRICAL_SURFACE('',#7413,12.375);
#6229=CYLINDRICAL_SURFACE('',#7414,0.269999999999999);
#6230=CYLINDRICAL_SURFACE('',#7415,3.68751484013274);
#6231=CYLINDRICAL_SURFACE('',#7416,3.68751484013274);
#6232=CYLINDRICAL_SURFACE('',#7417,0.269999999999999);
#6233=CYLINDRICAL_SURFACE('',#7418,12.375);
#6234=CYLINDRICAL_SURFACE('',#7419,0.269999999999999);
#6235=CYLINDRICAL_SURFACE('',#7420,3.68751484013274);
#6236=CYLINDRICAL_SURFACE('',#7421,3.68751484013274);
#6237=CYLINDRICAL_SURFACE('',#7422,0.269999999999999);
#6238=CYLINDRICAL_SURFACE('',#7423,12.375);
#6239=CYLINDRICAL_SURFACE('',#7424,0.269999999999999);
#6240=CYLINDRICAL_SURFACE('',#7425,3.68751484013274);
#6241=CYLINDRICAL_SURFACE('',#7426,3.68751484013274);
#6242=CYLINDRICAL_SURFACE('',#7427,0.269999999999999);
#6243=CYLINDRICAL_SURFACE('',#7428,12.375);
#6244=CYLINDRICAL_SURFACE('',#7429,0.269999999999999);
#6245=CYLINDRICAL_SURFACE('',#7430,3.68751484013274);
#6246=CYLINDRICAL_SURFACE('',#7431,3.68751484013274);
#6247=CYLINDRICAL_SURFACE('',#7432,0.269999999999999);
#6248=CYLINDRICAL_SURFACE('',#7433,12.375);
#6249=CYLINDRICAL_SURFACE('',#7434,0.269999999999999);
#6250=CYLINDRICAL_SURFACE('',#7435,3.68751484013274);
#6251=CYLINDRICAL_SURFACE('',#7436,3.68751484013274);
#6252=CYLINDRICAL_SURFACE('',#7437,0.269999999999999);
#6253=CYLINDRICAL_SURFACE('',#7438,12.375);
#6254=CYLINDRICAL_SURFACE('',#7439,0.269999999999999);
#6255=CYLINDRICAL_SURFACE('',#7440,3.68751484013274);
#6256=CYLINDRICAL_SURFACE('',#7441,3.68751484013274);
#6257=CYLINDRICAL_SURFACE('',#7442,0.269999999999999);
#6258=CYLINDRICAL_SURFACE('',#7443,12.375);
#6259=CYLINDRICAL_SURFACE('',#7444,0.269999999999999);
#6364=ADVANCED_FACE('',(#394),#6079,.F.);
#6365=ADVANCED_FACE('',(#395),#6080,.F.);
#6366=ADVANCED_FACE('',(#396),#6081,.T.);
#6367=ADVANCED_FACE('',(#397),#6082,.F.);
#6368=ADVANCED_FACE('',(#398),#6083,.T.);
#6369=ADVANCED_FACE('',(#399),#6084,.F.);
#6370=ADVANCED_FACE('',(#400),#6085,.T.);
#6371=ADVANCED_FACE('',(#401),#6086,.F.);
#6372=ADVANCED_FACE('',(#402),#6087,.T.);
#6373=ADVANCED_FACE('',(#403),#6088,.F.);
#6374=ADVANCED_FACE('',(#404),#6089,.F.);
#6375=ADVANCED_FACE('',(#405),#6090,.F.);
#6376=ADVANCED_FACE('',(#406),#6091,.F.);
#6377=ADVANCED_FACE('',(#407),#6092,.F.);
#6378=ADVANCED_FACE('',(#408),#6093,.F.);
#6379=ADVANCED_FACE('',(#409),#6094,.F.);
#6380=ADVANCED_FACE('',(#410),#6095,.F.);
#6381=ADVANCED_FACE('',(#411),#6096,.F.);
#6382=ADVANCED_FACE('',(#412),#6097,.F.);
#6383=ADVANCED_FACE('',(#413),#6098,.T.);
#6384=ADVANCED_FACE('',(#414),#6099,.T.);
#6385=ADVANCED_FACE('',(#415),#6100,.T.);
#6386=ADVANCED_FACE('',(#416),#6101,.T.);
#6387=ADVANCED_FACE('',(#417),#6102,.T.);
#6388=ADVANCED_FACE('',(#418),#6103,.T.);
#6389=ADVANCED_FACE('',(#419),#6104,.T.);
#6390=ADVANCED_FACE('',(#420),#6105,.T.);
#6391=ADVANCED_FACE('',(#421),#6106,.T.);
#6392=ADVANCED_FACE('',(#422),#6107,.T.);
#6393=ADVANCED_FACE('',(#423),#6108,.T.);
#6394=ADVANCED_FACE('',(#424),#6109,.T.);
#6395=ADVANCED_FACE('',(#425),#6110,.T.);
#6396=ADVANCED_FACE('',(#426),#6111,.T.);
#6397=ADVANCED_FACE('',(#427),#6112,.T.);
#6398=ADVANCED_FACE('',(#428),#6113,.T.);
#6399=ADVANCED_FACE('',(#429),#6114,.T.);
#6400=ADVANCED_FACE('',(#430),#6115,.T.);
#6401=ADVANCED_FACE('',(#431),#6116,.T.);
#6402=ADVANCED_FACE('',(#432),#6117,.T.);
#6403=ADVANCED_FACE('',(#433),#6118,.T.);
#6404=ADVANCED_FACE('',(#434),#6119,.T.);
#6405=ADVANCED_FACE('',(#435),#6120,.T.);
#6406=ADVANCED_FACE('',(#436),#6121,.T.);
#6407=ADVANCED_FACE('',(#437),#6122,.T.);
#6408=ADVANCED_FACE('',(#438),#6123,.T.);
#6409=ADVANCED_FACE('',(#439),#6124,.T.);
#6410=ADVANCED_FACE('',(#440),#6125,.T.);
#6411=ADVANCED_FACE('',(#441),#6126,.T.);
#6412=ADVANCED_FACE('',(#442,#192),#251,.F.);
#6413=ADVANCED_FACE('',(#443,#193),#252,.T.);
#6414=ADVANCED_FACE('',(#444),#6127,.T.);
#6415=ADVANCED_FACE('',(#445),#6128,.T.);
#6416=ADVANCED_FACE('',(#446),#6129,.T.);
#6417=ADVANCED_FACE('',(#447),#6130,.T.);
#6418=ADVANCED_FACE('',(#448),#6131,.F.);
#6419=ADVANCED_FACE('',(#449),#6132,.F.);
#6420=ADVANCED_FACE('',(#450),#6133,.T.);
#6421=ADVANCED_FACE('',(#451),#6134,.T.);
#6422=ADVANCED_FACE('',(#452),#6135,.F.);
#6423=ADVANCED_FACE('',(#453),#6136,.T.);
#6424=ADVANCED_FACE('',(#454),#6137,.F.);
#6425=ADVANCED_FACE('',(#455),#6138,.T.);
#6426=ADVANCED_FACE('',(#456),#6139,.T.);
#6427=ADVANCED_FACE('',(#457),#6140,.F.);
#6428=ADVANCED_FACE('',(#458),#6141,.T.);
#6429=ADVANCED_FACE('',(#459),#6142,.T.);
#6430=ADVANCED_FACE('',(#460),#6143,.T.);
#6431=ADVANCED_FACE('',(#461),#6144,.F.);
#6432=ADVANCED_FACE('',(#462),#6145,.T.);
#6433=ADVANCED_FACE('',(#463),#6146,.T.);
#6434=ADVANCED_FACE('',(#464),#6147,.T.);
#6435=ADVANCED_FACE('',(#465),#6148,.F.);
#6436=ADVANCED_FACE('',(#466),#6149,.T.);
#6437=ADVANCED_FACE('',(#467),#6150,.T.);
#6438=ADVANCED_FACE('',(#468),#6151,.T.);
#6439=ADVANCED_FACE('',(#469),#6152,.F.);
#6440=ADVANCED_FACE('',(#470),#6153,.T.);
#6441=ADVANCED_FACE('',(#471),#6154,.T.);
#6442=ADVANCED_FACE('',(#472),#6155,.T.);
#6443=ADVANCED_FACE('',(#473),#6156,.F.);
#6444=ADVANCED_FACE('',(#474),#6157,.T.);
#6445=ADVANCED_FACE('',(#475),#6158,.T.);
#6446=ADVANCED_FACE('',(#476),#6159,.T.);
#6447=ADVANCED_FACE('',(#477),#6160,.T.);
#6448=ADVANCED_FACE('',(#478),#6161,.F.);
#6449=ADVANCED_FACE('',(#479),#6162,.T.);
#6450=ADVANCED_FACE('',(#480),#6163,.T.);
#6451=ADVANCED_FACE('',(#481),#6164,.T.);
#6452=ADVANCED_FACE('',(#482),#6165,.F.);
#6453=ADVANCED_FACE('',(#483),#6166,.T.);
#6454=ADVANCED_FACE('',(#484),#6167,.T.);
#6455=ADVANCED_FACE('',(#485),#6168,.T.);
#6456=ADVANCED_FACE('',(#486),#6169,.F.);
#6457=ADVANCED_FACE('',(#487),#6170,.T.);
#6458=ADVANCED_FACE('',(#488),#6171,.T.);
#6459=ADVANCED_FACE('',(#489),#6172,.T.);
#6460=ADVANCED_FACE('',(#490),#6173,.F.);
#6461=ADVANCED_FACE('',(#491),#6174,.T.);
#6462=ADVANCED_FACE('',(#492),#6175,.T.);
#6463=ADVANCED_FACE('',(#493),#6176,.T.);
#6464=ADVANCED_FACE('',(#494),#6177,.F.);
#6465=ADVANCED_FACE('',(#495),#6178,.T.);
#6466=ADVANCED_FACE('',(#496),#6179,.T.);
#6467=ADVANCED_FACE('',(#497),#6180,.F.);
#6468=ADVANCED_FACE('',(#498),#6181,.T.);
#6469=ADVANCED_FACE('',(#499),#6182,.T.);
#6470=ADVANCED_FACE('',(#500),#6183,.F.);
#6471=ADVANCED_FACE('',(#501),#6184,.T.);
#6472=ADVANCED_FACE('',(#502),#6185,.F.);
#6473=ADVANCED_FACE('',(#503),#6186,.T.);
#6474=ADVANCED_FACE('',(#504),#6187,.T.);
#6475=ADVANCED_FACE('',(#505),#6188,.F.);
#6476=ADVANCED_FACE('',(#506),#6189,.T.);
#6477=ADVANCED_FACE('',(#507),#6190,.T.);
#6478=ADVANCED_FACE('',(#508),#6191,.T.);
#6479=ADVANCED_FACE('',(#509),#6192,.F.);
#6480=ADVANCED_FACE('',(#510),#6193,.T.);
#6481=ADVANCED_FACE('',(#511),#6194,.F.);
#6482=ADVANCED_FACE('',(#512),#6195,.T.);
#6483=ADVANCED_FACE('',(#513),#6196,.T.);
#6484=ADVANCED_FACE('',(#514),#6197,.F.);
#6485=ADVANCED_FACE('',(#515),#6198,.T.);
#6486=ADVANCED_FACE('',(#516),#6199,.F.);
#6487=ADVANCED_FACE('',(#517),#6200,.T.);
#6488=ADVANCED_FACE('',(#518),#6201,.T.);
#6489=ADVANCED_FACE('',(#519),#6202,.F.);
#6490=ADVANCED_FACE('',(#520),#6203,.T.);
#6491=ADVANCED_FACE('',(#521),#6204,.F.);
#6492=ADVANCED_FACE('',(#522),#6205,.T.);
#6493=ADVANCED_FACE('',(#523),#6206,.T.);
#6494=ADVANCED_FACE('',(#524),#6207,.F.);
#6495=ADVANCED_FACE('',(#525),#6208,.T.);
#6496=ADVANCED_FACE('',(#526),#6209,.F.);
#6497=ADVANCED_FACE('',(#527),#6210,.T.);
#6498=ADVANCED_FACE('',(#528),#6211,.T.);
#6499=ADVANCED_FACE('',(#529),#6212,.F.);
#6500=ADVANCED_FACE('',(#530),#6213,.T.);
#6501=ADVANCED_FACE('',(#531),#6214,.F.);
#6502=ADVANCED_FACE('',(#532),#6215,.T.);
#6503=ADVANCED_FACE('',(#533),#6216,.T.);
#6504=ADVANCED_FACE('',(#534),#6217,.F.);
#6505=ADVANCED_FACE('',(#535),#6218,.T.);
#6506=ADVANCED_FACE('',(#536),#6219,.F.);
#6507=ADVANCED_FACE('',(#537),#6220,.T.);
#6508=ADVANCED_FACE('',(#538),#6221,.T.);
#6509=ADVANCED_FACE('',(#539),#6222,.F.);
#6510=ADVANCED_FACE('',(#540),#6223,.T.);
#6511=ADVANCED_FACE('',(#541),#6224,.F.);
#6512=ADVANCED_FACE('',(#542),#6225,.T.);
#6513=ADVANCED_FACE('',(#543),#6226,.T.);
#6514=ADVANCED_FACE('',(#544),#6227,.F.);
#6515=ADVANCED_FACE('',(#545),#6228,.T.);
#6516=ADVANCED_FACE('',(#546),#6229,.F.);
#6517=ADVANCED_FACE('',(#547),#6230,.T.);
#6518=ADVANCED_FACE('',(#548),#6231,.T.);
#6519=ADVANCED_FACE('',(#549),#6232,.F.);
#6520=ADVANCED_FACE('',(#550),#6233,.T.);
#6521=ADVANCED_FACE('',(#551),#6234,.F.);
#6522=ADVANCED_FACE('',(#552),#6235,.T.);
#6523=ADVANCED_FACE('',(#553),#6236,.T.);
#6524=ADVANCED_FACE('',(#554),#6237,.F.);
#6525=ADVANCED_FACE('',(#555),#6238,.T.);
#6526=ADVANCED_FACE('',(#556),#6239,.F.);
#6527=ADVANCED_FACE('',(#557),#6240,.T.);
#6528=ADVANCED_FACE('',(#558),#6241,.T.);
#6529=ADVANCED_FACE('',(#559),#6242,.F.);
#6530=ADVANCED_FACE('',(#560),#6243,.T.);
#6531=ADVANCED_FACE('',(#561),#6244,.F.);
#6532=ADVANCED_FACE('',(#562),#6245,.T.);
#6533=ADVANCED_FACE('',(#563),#6246,.T.);
#6534=ADVANCED_FACE('',(#564),#6247,.F.);
#6535=ADVANCED_FACE('',(#565),#6248,.T.);
#6536=ADVANCED_FACE('',(#566),#6249,.F.);
#6537=ADVANCED_FACE('',(#567),#6250,.T.);
#6538=ADVANCED_FACE('',(#568),#6251,.T.);
#6539=ADVANCED_FACE('',(#569),#6252,.F.);
#6540=ADVANCED_FACE('',(#570),#6253,.T.);
#6541=ADVANCED_FACE('',(#571),#6254,.F.);
#6542=ADVANCED_FACE('',(#572),#6255,.T.);
#6543=ADVANCED_FACE('',(#573),#6256,.T.);
#6544=ADVANCED_FACE('',(#574),#6257,.F.);
#6545=ADVANCED_FACE('',(#575),#6258,.T.);
#6546=ADVANCED_FACE('',(#576),#6259,.F.);
#6547=ADVANCED_FACE('',(#577),#253,.F.);
#6548=ADVANCED_FACE('',(#578),#254,.F.);
#6549=ADVANCED_FACE('',(#579),#255,.F.);
#6646=CLOSED_SHELL('',(#6364,#6365,#6366,#6367,#6368,#6369,#6370,#6371,
#6372,#6373,#6374,#6375,#6376,#6377,#6378,#6379,#6380,#6381,#6382,#6383,
#6384,#6385,#6386,#6387,#6388,#6389,#6390,#6391,#6392,#6393,#6394,#6395,
#6396,#6397,#6398,#6399,#6400,#6401,#6402,#6403,#6404,#6405,#6406,#6407,
#6408,#6409,#6410,#6411,#6412,#6413,#6414,#6415,#6416,#6417,#6418,#6419,
#6420,#6421,#6422,#6423,#6424,#6425,#6426,#6427,#6428,#6429,#6430,#6431,
#6432,#6433,#6434,#6435,#6436,#6437,#6438,#6439,#6440,#6441,#6442,#6443,
#6444,#6445,#6446,#6447,#6448,#6449,#6450,#6451,#6452,#6453,#6454,#6455,
#6456,#6457,#6458,#6459,#6460,#6461,#6462,#6463,#6464,#6465,#6466,#6467,
#6468,#6469,#6470,#6471,#6472,#6473,#6474,#6475,#6476,#6477,#6478,#6479,
#6480,#6481,#6482,#6483,#6484,#6485,#6486,#6487,#6488,#6489,#6490,#6491,
#6492,#6493,#6494,#6495,#6496,#6497,#6498,#6499,#6500,#6501,#6502,#6503,
#6504,#6505,#6506,#6507,#6508,#6509,#6510,#6511,#6512,#6513,#6514,#6515,
#6516,#6517,#6518,#6519,#6520,#6521,#6522,#6523,#6524,#6525,#6526,#6527,
#6528,#6529,#6530,#6531,#6532,#6533,#6534,#6535,#6536,#6537,#6538,#6539,
#6540,#6541,#6542,#6543,#6544,#6545,#6546,#6547,#6548,#6549));
#6899=AXIS2_PLACEMENT_3D('',#10298,#8063,#8064);
#6900=AXIS2_PLACEMENT_3D('',#10299,#8065,#8066);
#6901=AXIS2_PLACEMENT_3D('',#10302,#8067,#8068);
#6902=AXIS2_PLACEMENT_3D('',#10306,#8070,#8071);
#6903=AXIS2_PLACEMENT_3D('',#10308,#8073,#8074);
#6904=AXIS2_PLACEMENT_3D('',#10311,#8075,#8076);
#6905=AXIS2_PLACEMENT_3D('',#10315,#8078,#8079);
#6906=AXIS2_PLACEMENT_3D('',#10317,#8081,#8082);
#6907=AXIS2_PLACEMENT_3D('',#10319,#8083,#8084);
#6908=AXIS2_PLACEMENT_3D('',#10322,#8086,#8087);
#6909=AXIS2_PLACEMENT_3D('',#10323,#8088,#8089);
#6910=AXIS2_PLACEMENT_3D('',#10326,#8090,#8091);
#6911=AXIS2_PLACEMENT_3D('',#10330,#8093,#8094);
#6912=AXIS2_PLACEMENT_3D('',#10332,#8096,#8097);
#6913=AXIS2_PLACEMENT_3D('',#10334,#8098,#8099);
#6914=AXIS2_PLACEMENT_3D('',#10337,#8101,#8102);
#6915=AXIS2_PLACEMENT_3D('',#10338,#8103,#8104);
#6916=AXIS2_PLACEMENT_3D('',#10341,#8105,#8106);
#6917=AXIS2_PLACEMENT_3D('',#10345,#8108,#8109);
#6918=AXIS2_PLACEMENT_3D('',#10347,#8111,#8112);
#6919=AXIS2_PLACEMENT_3D('',#10349,#8113,#8114);
#6920=AXIS2_PLACEMENT_3D('',#10351,#8115,#8116);
#6921=AXIS2_PLACEMENT_3D('',#10353,#8118,#8119);
#6922=AXIS2_PLACEMENT_3D('',#10356,#8120,#8121);
#6923=AXIS2_PLACEMENT_3D('',#10360,#8123,#8124);
#6924=AXIS2_PLACEMENT_3D('',#10362,#8126,#8127);
#6925=AXIS2_PLACEMENT_3D('',#10364,#8128,#8129);
#6926=AXIS2_PLACEMENT_3D('',#10366,#8130,#8131);
#6927=AXIS2_PLACEMENT_3D('',#10368,#8133,#8134);
#6928=AXIS2_PLACEMENT_3D('',#10371,#8135,#8136);
#6929=AXIS2_PLACEMENT_3D('',#10375,#8138,#8139);
#6930=AXIS2_PLACEMENT_3D('',#10377,#8141,#8142);
#6931=AXIS2_PLACEMENT_3D('',#10380,#8143,#8144);
#6932=AXIS2_PLACEMENT_3D('',#10384,#8146,#8147);
#6933=AXIS2_PLACEMENT_3D('',#10386,#8149,#8150);
#6934=AXIS2_PLACEMENT_3D('',#10389,#8151,#8152);
#6935=AXIS2_PLACEMENT_3D('',#10393,#8154,#8155);
#6936=AXIS2_PLACEMENT_3D('',#10395,#8157,#8158);
#6937=AXIS2_PLACEMENT_3D('',#10398,#8159,#8160);
#6938=AXIS2_PLACEMENT_3D('',#10402,#8162,#8163);
#6939=AXIS2_PLACEMENT_3D('',#10404,#8165,#8166);
#6940=AXIS2_PLACEMENT_3D('',#10407,#8167,#8168);
#6941=AXIS2_PLACEMENT_3D('',#10411,#8170,#8171);
#6942=AXIS2_PLACEMENT_3D('',#10413,#8173,#8174);
#6943=AXIS2_PLACEMENT_3D('',#10416,#8175,#8176);
#6944=AXIS2_PLACEMENT_3D('',#10420,#8178,#8179);
#6945=AXIS2_PLACEMENT_3D('',#10422,#8181,#8182);
#6946=AXIS2_PLACEMENT_3D('',#10425,#8183,#8184);
#6947=AXIS2_PLACEMENT_3D('',#10429,#8186,#8187);
#6948=AXIS2_PLACEMENT_3D('',#10431,#8189,#8190);
#6949=AXIS2_PLACEMENT_3D('',#10434,#8191,#8192);
#6950=AXIS2_PLACEMENT_3D('',#10438,#8194,#8195);
#6951=AXIS2_PLACEMENT_3D('',#10440,#8197,#8198);
#6952=AXIS2_PLACEMENT_3D('',#10443,#8199,#8200);
#6953=AXIS2_PLACEMENT_3D('',#10447,#8202,#8203);
#6954=AXIS2_PLACEMENT_3D('',#10449,#8205,#8206);
#6955=AXIS2_PLACEMENT_3D('',#10452,#8207,#8208);
#6956=AXIS2_PLACEMENT_3D('',#10456,#8210,#8211);
#6957=AXIS2_PLACEMENT_3D('',#10458,#8213,#8214);
#6958=AXIS2_PLACEMENT_3D('',#10461,#8215,#8216);
#6959=AXIS2_PLACEMENT_3D('',#10465,#8218,#8219);
#6960=AXIS2_PLACEMENT_3D('',#10467,#8221,#8222);
#6961=AXIS2_PLACEMENT_3D('',#10470,#8223,#8224);
#6962=AXIS2_PLACEMENT_3D('',#10474,#8226,#8227);
#6963=AXIS2_PLACEMENT_3D('',#10476,#8229,#8230);
#6964=AXIS2_PLACEMENT_3D('',#10479,#8231,#8232);
#6965=AXIS2_PLACEMENT_3D('',#10483,#8234,#8235);
#6966=AXIS2_PLACEMENT_3D('',#10485,#8237,#8238);
#6967=AXIS2_PLACEMENT_3D('',#10488,#8239,#8240);
#6968=AXIS2_PLACEMENT_3D('',#10492,#8242,#8243);
#6969=AXIS2_PLACEMENT_3D('',#10494,#8245,#8246);
#6970=AXIS2_PLACEMENT_3D('',#10497,#8247,#8248);
#6971=AXIS2_PLACEMENT_3D('',#10501,#8250,#8251);
#6972=AXIS2_PLACEMENT_3D('',#10503,#8253,#8254);
#6973=AXIS2_PLACEMENT_3D('',#10506,#8255,#8256);
#6974=AXIS2_PLACEMENT_3D('',#10510,#8258,#8259);
#6975=AXIS2_PLACEMENT_3D('',#10512,#8261,#8262);
#6976=AXIS2_PLACEMENT_3D('',#10515,#8263,#8264);
#6977=AXIS2_PLACEMENT_3D('',#10519,#8266,#8267);
#6978=AXIS2_PLACEMENT_3D('',#10521,#8269,#8270);
#6979=AXIS2_PLACEMENT_3D('',#10524,#8271,#8272);
#6980=AXIS2_PLACEMENT_3D('',#10528,#8274,#8275);
#6981=AXIS2_PLACEMENT_3D('',#10530,#8277,#8278);
#6982=AXIS2_PLACEMENT_3D('',#10533,#8279,#8280);
#6983=AXIS2_PLACEMENT_3D('',#10537,#8282,#8283);
#6984=AXIS2_PLACEMENT_3D('',#10539,#8285,#8286);
#6985=AXIS2_PLACEMENT_3D('',#10542,#8287,#8288);
#6986=AXIS2_PLACEMENT_3D('',#10546,#8290,#8291);
#6987=AXIS2_PLACEMENT_3D('',#10548,#8293,#8294);
#6988=AXIS2_PLACEMENT_3D('',#10551,#8295,#8296);
#6989=AXIS2_PLACEMENT_3D('',#10555,#8298,#8299);
#6990=AXIS2_PLACEMENT_3D('',#10557,#8301,#8302);
#6991=AXIS2_PLACEMENT_3D('',#10560,#8303,#8304);
#6992=AXIS2_PLACEMENT_3D('',#10564,#8306,#8307);
#6993=AXIS2_PLACEMENT_3D('',#10566,#8309,#8310);
#6994=AXIS2_PLACEMENT_3D('',#10569,#8311,#8312);
#6995=AXIS2_PLACEMENT_3D('',#10573,#8314,#8315);
#6996=AXIS2_PLACEMENT_3D('',#10575,#8317,#8318);
#6997=AXIS2_PLACEMENT_3D('',#10578,#8319,#8320);
#6998=AXIS2_PLACEMENT_3D('',#10582,#8322,#8323);
#6999=AXIS2_PLACEMENT_3D('',#10584,#8325,#8326);
#7000=AXIS2_PLACEMENT_3D('',#10586,#8327,#8328);
#7001=AXIS2_PLACEMENT_3D('',#10589,#8330,#8331);
#7002=AXIS2_PLACEMENT_3D('',#10590,#8332,#8333);
#7003=AXIS2_PLACEMENT_3D('',#10592,#8334,#8335);
#7004=AXIS2_PLACEMENT_3D('',#10595,#8337,#8338);
#7005=AXIS2_PLACEMENT_3D('',#10596,#8339,#8340);
#7006=AXIS2_PLACEMENT_3D('',#10598,#8341,#8342);
#7007=AXIS2_PLACEMENT_3D('',#10601,#8344,#8345);
#7008=AXIS2_PLACEMENT_3D('',#10602,#8346,#8347);
#7009=AXIS2_PLACEMENT_3D('',#10605,#8348,#8349);
#7010=AXIS2_PLACEMENT_3D('',#10609,#8351,#8352);
#7011=AXIS2_PLACEMENT_3D('',#10611,#8354,#8355);
#7012=AXIS2_PLACEMENT_3D('',#10614,#8356,#8357);
#7013=AXIS2_PLACEMENT_3D('',#10618,#8359,#8360);
#7014=AXIS2_PLACEMENT_3D('',#10620,#8362,#8363);
#7015=AXIS2_PLACEMENT_3D('',#10623,#8364,#8365);
#7016=AXIS2_PLACEMENT_3D('',#10627,#8367,#8368);
#7017=AXIS2_PLACEMENT_3D('',#10629,#8370,#8371);
#7018=AXIS2_PLACEMENT_3D('',#10632,#8372,#8373);
#7019=AXIS2_PLACEMENT_3D('',#10636,#8375,#8376);
#7020=AXIS2_PLACEMENT_3D('',#10638,#8378,#8379);
#7021=AXIS2_PLACEMENT_3D('',#10641,#8380,#8381);
#7022=AXIS2_PLACEMENT_3D('',#10645,#8383,#8384);
#7023=AXIS2_PLACEMENT_3D('',#10647,#8386,#8387);
#7024=AXIS2_PLACEMENT_3D('',#10650,#8388,#8389);
#7025=AXIS2_PLACEMENT_3D('',#10654,#8391,#8392);
#7026=AXIS2_PLACEMENT_3D('',#10656,#8394,#8395);
#7027=AXIS2_PLACEMENT_3D('',#10659,#8396,#8397);
#7028=AXIS2_PLACEMENT_3D('',#10663,#8399,#8400);
#7029=AXIS2_PLACEMENT_3D('',#10665,#8402,#8403);
#7030=AXIS2_PLACEMENT_3D('',#10668,#8404,#8405);
#7031=AXIS2_PLACEMENT_3D('',#10672,#8407,#8408);
#7032=AXIS2_PLACEMENT_3D('',#10674,#8410,#8411);
#7033=AXIS2_PLACEMENT_3D('',#10677,#8412,#8413);
#7034=AXIS2_PLACEMENT_3D('',#10681,#8415,#8416);
#7035=AXIS2_PLACEMENT_3D('',#10683,#8418,#8419);
#7036=AXIS2_PLACEMENT_3D('',#10686,#8420,#8421);
#7037=AXIS2_PLACEMENT_3D('',#10690,#8423,#8424);
#7038=AXIS2_PLACEMENT_3D('',#10692,#8426,#8427);
#7039=AXIS2_PLACEMENT_3D('',#10695,#8428,#8429);
#7040=AXIS2_PLACEMENT_3D('',#10699,#8431,#8432);
#7041=AXIS2_PLACEMENT_3D('',#10701,#8434,#8435);
#7042=AXIS2_PLACEMENT_3D('',#10704,#8436,#8437);
#7043=AXIS2_PLACEMENT_3D('',#10708,#8439,#8440);
#7044=AXIS2_PLACEMENT_3D('',#10710,#8442,#8443);
#7045=AXIS2_PLACEMENT_3D('',#10712,#8444,#8445);
#7046=AXIS2_PLACEMENT_3D('',#10714,#8446,#8447);
#7047=AXIS2_PLACEMENT_3D('',#10716,#8448,#8449);
#7048=AXIS2_PLACEMENT_3D('',#10718,#8450,#8451);
#7049=AXIS2_PLACEMENT_3D('',#10719,#8452,#8453);
#7050=AXIS2_PLACEMENT_3D('',#10721,#8454,#8455);
#7051=AXIS2_PLACEMENT_3D('',#10723,#8456,#8457);
#7052=AXIS2_PLACEMENT_3D('',#10725,#8458,#8459);
#7053=AXIS2_PLACEMENT_3D('',#10727,#8460,#8461);
#7054=AXIS2_PLACEMENT_3D('',#10728,#8462,#8463);
#7055=AXIS2_PLACEMENT_3D('',#10730,#8464,#8465);
#7056=AXIS2_PLACEMENT_3D('',#10732,#8466,#8467);
#7057=AXIS2_PLACEMENT_3D('',#10734,#8468,#8469);
#7058=AXIS2_PLACEMENT_3D('',#10736,#8470,#8471);
#7059=AXIS2_PLACEMENT_3D('',#10737,#8472,#8473);
#7060=AXIS2_PLACEMENT_3D('',#10739,#8474,#8475);
#7061=AXIS2_PLACEMENT_3D('',#10741,#8476,#8477);
#7062=AXIS2_PLACEMENT_3D('',#10743,#8478,#8479);
#7063=AXIS2_PLACEMENT_3D('',#10745,#8480,#8481);
#7064=AXIS2_PLACEMENT_3D('',#10746,#8482,#8483);
#7065=AXIS2_PLACEMENT_3D('',#10748,#8484,#8485);
#7066=AXIS2_PLACEMENT_3D('',#10750,#8486,#8487);
#7067=AXIS2_PLACEMENT_3D('',#10752,#8488,#8489);
#7068=AXIS2_PLACEMENT_3D('',#10754,#8490,#8491);
#7069=AXIS2_PLACEMENT_3D('',#10755,#8492,#8493);
#7070=AXIS2_PLACEMENT_3D('',#10757,#8494,#8495);
#7071=AXIS2_PLACEMENT_3D('',#10759,#8496,#8497);
#7072=AXIS2_PLACEMENT_3D('',#10761,#8498,#8499);
#7073=AXIS2_PLACEMENT_3D('',#10763,#8500,#8501);
#7074=AXIS2_PLACEMENT_3D('',#10764,#8502,#8503);
#7075=AXIS2_PLACEMENT_3D('',#10766,#8504,#8505);
#7076=AXIS2_PLACEMENT_3D('',#10768,#8506,#8507);
#7077=AXIS2_PLACEMENT_3D('',#10770,#8508,#8509);
#7078=AXIS2_PLACEMENT_3D('',#10772,#8510,#8511);
#7079=AXIS2_PLACEMENT_3D('',#10773,#8512,#8513);
#7080=AXIS2_PLACEMENT_3D('',#10775,#8514,#8515);
#7081=AXIS2_PLACEMENT_3D('',#10777,#8516,#8517);
#7082=AXIS2_PLACEMENT_3D('',#10779,#8518,#8519);
#7083=AXIS2_PLACEMENT_3D('',#10781,#8520,#8521);
#7084=AXIS2_PLACEMENT_3D('',#10782,#8522,#8523);
#7085=AXIS2_PLACEMENT_3D('',#10784,#8524,#8525);
#7086=AXIS2_PLACEMENT_3D('',#10786,#8526,#8527);
#7087=AXIS2_PLACEMENT_3D('',#10788,#8528,#8529);
#7088=AXIS2_PLACEMENT_3D('',#10790,#8530,#8531);
#7089=AXIS2_PLACEMENT_3D('',#10791,#8532,#8533);
#7090=AXIS2_PLACEMENT_3D('',#10793,#8534,#8535);
#7091=AXIS2_PLACEMENT_3D('',#10795,#8536,#8537);
#7092=AXIS2_PLACEMENT_3D('',#10797,#8538,#8539);
#7093=AXIS2_PLACEMENT_3D('',#10799,#8540,#8541);
#7094=AXIS2_PLACEMENT_3D('',#10800,#8542,#8543);
#7095=AXIS2_PLACEMENT_3D('',#10802,#8544,#8545);
#7096=AXIS2_PLACEMENT_3D('',#10804,#8546,#8547);
#7097=AXIS2_PLACEMENT_3D('',#10806,#8548,#8549);
#7098=AXIS2_PLACEMENT_3D('',#10808,#8550,#8551);
#7099=AXIS2_PLACEMENT_3D('',#10809,#8552,#8553);
#7100=AXIS2_PLACEMENT_3D('',#10811,#8554,#8555);
#7101=AXIS2_PLACEMENT_3D('',#10813,#8556,#8557);
#7102=AXIS2_PLACEMENT_3D('',#10815,#8558,#8559);
#7103=AXIS2_PLACEMENT_3D('',#10817,#8560,#8561);
#7104=AXIS2_PLACEMENT_3D('',#10818,#8562,#8563);
#7105=AXIS2_PLACEMENT_3D('',#10820,#8564,#8565);
#7106=AXIS2_PLACEMENT_3D('',#10822,#8566,#8567);
#7107=AXIS2_PLACEMENT_3D('',#10823,#8568,#8569);
#7108=AXIS2_PLACEMENT_3D('',#10825,#8570,#8571);
#7109=AXIS2_PLACEMENT_3D('',#10827,#8572,#8573);
#7110=AXIS2_PLACEMENT_3D('',#10828,#8574,#8575);
#7111=AXIS2_PLACEMENT_3D('',#10829,#8576,#8577);
#7112=AXIS2_PLACEMENT_3D('',#10831,#8578,#8579);
#7113=AXIS2_PLACEMENT_3D('',#10833,#8580,#8581);
#7114=AXIS2_PLACEMENT_3D('',#10834,#8582,#8583);
#7115=AXIS2_PLACEMENT_3D('',#10835,#8584,#8585);
#7116=AXIS2_PLACEMENT_3D('',#10837,#8586,#8587);
#7117=AXIS2_PLACEMENT_3D('',#10839,#8588,#8589);
#7118=AXIS2_PLACEMENT_3D('',#10840,#8590,#8591);
#7119=AXIS2_PLACEMENT_3D('',#10841,#8592,#8593);
#7120=AXIS2_PLACEMENT_3D('',#10843,#8594,#8595);
#7121=AXIS2_PLACEMENT_3D('',#10845,#8596,#8597);
#7122=AXIS2_PLACEMENT_3D('',#10846,#8598,#8599);
#7123=AXIS2_PLACEMENT_3D('',#10847,#8600,#8601);
#7124=AXIS2_PLACEMENT_3D('',#10849,#8602,#8603);
#7125=AXIS2_PLACEMENT_3D('',#10851,#8604,#8605);
#7126=AXIS2_PLACEMENT_3D('',#10852,#8606,#8607);
#7127=AXIS2_PLACEMENT_3D('',#10853,#8608,#8609);
#7128=AXIS2_PLACEMENT_3D('',#10855,#8610,#8611);
#7129=AXIS2_PLACEMENT_3D('',#10857,#8612,#8613);
#7130=AXIS2_PLACEMENT_3D('',#10858,#8614,#8615);
#7131=AXIS2_PLACEMENT_3D('',#10860,#8616,#8617);
#7132=AXIS2_PLACEMENT_3D('',#10862,#8618,#8619);
#7133=AXIS2_PLACEMENT_3D('',#10863,#8620,#8621);
#7134=AXIS2_PLACEMENT_3D('',#10864,#8622,#8623);
#7135=AXIS2_PLACEMENT_3D('',#10866,#8624,#8625);
#7136=AXIS2_PLACEMENT_3D('',#10868,#8626,#8627);
#7137=AXIS2_PLACEMENT_3D('',#10869,#8628,#8629);
#7138=AXIS2_PLACEMENT_3D('',#10870,#8630,#8631);
#7139=AXIS2_PLACEMENT_3D('',#10872,#8632,#8633);
#7140=AXIS2_PLACEMENT_3D('',#10874,#8634,#8635);
#7141=AXIS2_PLACEMENT_3D('',#10875,#8636,#8637);
#7142=AXIS2_PLACEMENT_3D('',#10876,#8638,#8639);
#7143=AXIS2_PLACEMENT_3D('',#10878,#8640,#8641);
#7144=AXIS2_PLACEMENT_3D('',#10880,#8642,#8643);
#7145=AXIS2_PLACEMENT_3D('',#10881,#8644,#8645);
#7146=AXIS2_PLACEMENT_3D('',#10882,#8646,#8647);
#7147=AXIS2_PLACEMENT_3D('',#10884,#8648,#8649);
#7148=AXIS2_PLACEMENT_3D('',#10886,#8650,#8651);
#7149=AXIS2_PLACEMENT_3D('',#10887,#8652,#8653);
#7150=AXIS2_PLACEMENT_3D('',#10888,#8654,#8655);
#7151=AXIS2_PLACEMENT_3D('',#10890,#8656,#8657);
#7152=AXIS2_PLACEMENT_3D('',#10892,#8658,#8659);
#7153=AXIS2_PLACEMENT_3D('',#10893,#8660,#8661);
#7154=AXIS2_PLACEMENT_3D('',#10895,#8662,#8663);
#7155=AXIS2_PLACEMENT_3D('',#10897,#8664,#8665);
#7156=AXIS2_PLACEMENT_3D('',#10898,#8666,#8667);
#7157=AXIS2_PLACEMENT_3D('',#10900,#8668,#8669);
#7158=AXIS2_PLACEMENT_3D('',#10902,#8670,#8671);
#7159=AXIS2_PLACEMENT_3D('',#10904,#8672,#8673);
#7160=AXIS2_PLACEMENT_3D('',#10906,#8674,#8675);
#7161=AXIS2_PLACEMENT_3D('',#10908,#8676,#8677);
#7162=AXIS2_PLACEMENT_3D('',#10909,#8678,#8679);
#7163=AXIS2_PLACEMENT_3D('',#10911,#8680,#8681);
#7164=AXIS2_PLACEMENT_3D('',#10913,#8682,#8683);
#7165=AXIS2_PLACEMENT_3D('',#10915,#8684,#8685);
#7166=AXIS2_PLACEMENT_3D('',#10917,#8686,#8687);
#7167=AXIS2_PLACEMENT_3D('',#10918,#8688,#8689);
#7168=AXIS2_PLACEMENT_3D('',#10920,#8690,#8691);
#7169=AXIS2_PLACEMENT_3D('',#10922,#8692,#8693);
#7170=AXIS2_PLACEMENT_3D('',#10924,#8694,#8695);
#7171=AXIS2_PLACEMENT_3D('',#10926,#8696,#8697);
#7172=AXIS2_PLACEMENT_3D('',#10927,#8698,#8699);
#7173=AXIS2_PLACEMENT_3D('',#10929,#8700,#8701);
#7174=AXIS2_PLACEMENT_3D('',#10931,#8702,#8703);
#7175=AXIS2_PLACEMENT_3D('',#10933,#8704,#8705);
#7176=AXIS2_PLACEMENT_3D('',#10935,#8706,#8707);
#7177=AXIS2_PLACEMENT_3D('',#10936,#8708,#8709);
#7178=AXIS2_PLACEMENT_3D('',#10942,#8713,#8714);
#7179=AXIS2_PLACEMENT_3D('',#10944,#8715,#8716);
#7180=AXIS2_PLACEMENT_3D('',#10946,#8717,#8718);
#7181=AXIS2_PLACEMENT_3D('',#10948,#8719,#8720);
#7182=AXIS2_PLACEMENT_3D('',#10950,#8721,#8722);
#7183=AXIS2_PLACEMENT_3D('',#10952,#8723,#8724);
#7184=AXIS2_PLACEMENT_3D('',#10953,#8725,#8726);
#7185=AXIS2_PLACEMENT_3D('',#10955,#8727,#8728);
#7186=AXIS2_PLACEMENT_3D('',#10957,#8729,#8730);
#7187=AXIS2_PLACEMENT_3D('',#10959,#8731,#8732);
#7188=AXIS2_PLACEMENT_3D('',#10961,#8733,#8734);
#7189=AXIS2_PLACEMENT_3D('',#10962,#8735,#8736);
#7190=AXIS2_PLACEMENT_3D('',#10964,#8737,#8738);
#7191=AXIS2_PLACEMENT_3D('',#10966,#8739,#8740);
#7192=AXIS2_PLACEMENT_3D('',#10968,#8741,#8742);
#7193=AXIS2_PLACEMENT_3D('',#10970,#8743,#8744);
#7194=AXIS2_PLACEMENT_3D('',#10971,#8745,#8746);
#7195=AXIS2_PLACEMENT_3D('',#10973,#8747,#8748);
#7196=AXIS2_PLACEMENT_3D('',#10975,#8749,#8750);
#7197=AXIS2_PLACEMENT_3D('',#10977,#8751,#8752);
#7198=AXIS2_PLACEMENT_3D('',#10979,#8753,#8754);
#7199=AXIS2_PLACEMENT_3D('',#10981,#8755,#8756);
#7200=AXIS2_PLACEMENT_3D('',#10982,#8757,#8758);
#7201=AXIS2_PLACEMENT_3D('',#10984,#8759,#8760);
#7202=AXIS2_PLACEMENT_3D('',#10986,#8761,#8762);
#7203=AXIS2_PLACEMENT_3D('',#10987,#8763,#8764);
#7204=AXIS2_PLACEMENT_3D('',#10989,#8765,#8766);
#7205=AXIS2_PLACEMENT_3D('',#10991,#8767,#8768);
#7206=AXIS2_PLACEMENT_3D('',#10992,#8769,#8770);
#7207=AXIS2_PLACEMENT_3D('',#10993,#8771,#8772);
#7208=AXIS2_PLACEMENT_3D('',#10995,#8773,#8774);
#7209=AXIS2_PLACEMENT_3D('',#10997,#8775,#8776);
#7210=AXIS2_PLACEMENT_3D('',#10998,#8777,#8778);
#7211=AXIS2_PLACEMENT_3D('',#10999,#8779,#8780);
#7212=AXIS2_PLACEMENT_3D('',#11001,#8781,#8782);
#7213=AXIS2_PLACEMENT_3D('',#11003,#8783,#8784);
#7214=AXIS2_PLACEMENT_3D('',#11004,#8785,#8786);
#7215=AXIS2_PLACEMENT_3D('',#11005,#8787,#8788);
#7216=AXIS2_PLACEMENT_3D('',#11007,#8789,#8790);
#7217=AXIS2_PLACEMENT_3D('',#11009,#8791,#8792);
#7218=AXIS2_PLACEMENT_3D('',#11010,#8793,#8794);
#7219=AXIS2_PLACEMENT_3D('',#11011,#8795,#8796);
#7220=AXIS2_PLACEMENT_3D('',#11013,#8797,#8798);
#7221=AXIS2_PLACEMENT_3D('',#11015,#8799,#8800);
#7222=AXIS2_PLACEMENT_3D('',#11016,#8801,#8802);
#7223=AXIS2_PLACEMENT_3D('',#11017,#8803,#8804);
#7224=AXIS2_PLACEMENT_3D('',#11019,#8805,#8806);
#7225=AXIS2_PLACEMENT_3D('',#11021,#8807,#8808);
#7226=AXIS2_PLACEMENT_3D('',#11022,#8809,#8810);
#7227=AXIS2_PLACEMENT_3D('',#11024,#8811,#8812);
#7228=AXIS2_PLACEMENT_3D('',#11026,#8813,#8814);
#7229=AXIS2_PLACEMENT_3D('',#11027,#8815,#8816);
#7230=AXIS2_PLACEMENT_3D('',#11028,#8817,#8818);
#7231=AXIS2_PLACEMENT_3D('',#11030,#8819,#8820);
#7232=AXIS2_PLACEMENT_3D('',#11032,#8821,#8822);
#7233=AXIS2_PLACEMENT_3D('',#11033,#8823,#8824);
#7234=AXIS2_PLACEMENT_3D('',#11034,#8825,#8826);
#7235=AXIS2_PLACEMENT_3D('',#11036,#8827,#8828);
#7236=AXIS2_PLACEMENT_3D('',#11038,#8829,#8830);
#7237=AXIS2_PLACEMENT_3D('',#11039,#8831,#8832);
#7238=AXIS2_PLACEMENT_3D('',#11040,#8833,#8834);
#7239=AXIS2_PLACEMENT_3D('',#11042,#8835,#8836);
#7240=AXIS2_PLACEMENT_3D('',#11044,#8837,#8838);
#7241=AXIS2_PLACEMENT_3D('',#11045,#8839,#8840);
#7242=AXIS2_PLACEMENT_3D('',#11046,#8841,#8842);
#7243=AXIS2_PLACEMENT_3D('',#11048,#8843,#8844);
#7244=AXIS2_PLACEMENT_3D('',#11050,#8845,#8846);
#7245=AXIS2_PLACEMENT_3D('',#11051,#8847,#8848);
#7246=AXIS2_PLACEMENT_3D('',#11052,#8849,#8850);
#7247=AXIS2_PLACEMENT_3D('',#11054,#8851,#8852);
#7248=AXIS2_PLACEMENT_3D('',#11056,#8853,#8854);
#7249=AXIS2_PLACEMENT_3D('',#11057,#8855,#8856);
#7250=AXIS2_PLACEMENT_3D('',#11059,#8857,#8858);
#7251=AXIS2_PLACEMENT_3D('',#11061,#8859,#8860);
#7252=AXIS2_PLACEMENT_3D('',#11062,#8861,#8862);
#7253=AXIS2_PLACEMENT_3D('',#11064,#8863,#8864);
#7254=AXIS2_PLACEMENT_3D('',#11066,#8865,#8866);
#7255=AXIS2_PLACEMENT_3D('',#11068,#8867,#8868);
#7256=AXIS2_PLACEMENT_3D('',#11070,#8869,#8870);
#7257=AXIS2_PLACEMENT_3D('',#11071,#8871,#8872);
#7258=AXIS2_PLACEMENT_3D('',#11073,#8873,#8874);
#7259=AXIS2_PLACEMENT_3D('',#11075,#8875,#8876);
#7260=AXIS2_PLACEMENT_3D('',#11077,#8877,#8878);
#7261=AXIS2_PLACEMENT_3D('',#11079,#8879,#8880);
#7262=AXIS2_PLACEMENT_3D('',#11080,#8881,#8882);
#7263=AXIS2_PLACEMENT_3D('',#11082,#8883,#8884);
#7264=AXIS2_PLACEMENT_3D('',#11084,#8885,#8886);
#7265=AXIS2_PLACEMENT_3D('',#11086,#8887,#8888);
#7266=AXIS2_PLACEMENT_3D('',#11088,#8889,#8890);
#7267=AXIS2_PLACEMENT_3D('',#11089,#8891,#8892);
#7268=AXIS2_PLACEMENT_3D('',#11091,#8893,#8894);
#7269=AXIS2_PLACEMENT_3D('',#11093,#8895,#8896);
#7270=AXIS2_PLACEMENT_3D('',#11095,#8897,#8898);
#7271=AXIS2_PLACEMENT_3D('',#11097,#8899,#8900);
#7272=AXIS2_PLACEMENT_3D('',#11098,#8901,#8902);
#7273=AXIS2_PLACEMENT_3D('',#11100,#8903,#8904);
#7274=AXIS2_PLACEMENT_3D('',#11102,#8905,#8906);
#7275=AXIS2_PLACEMENT_3D('',#11104,#8907,#8908);
#7276=AXIS2_PLACEMENT_3D('',#11106,#8909,#8910);
#7277=AXIS2_PLACEMENT_3D('',#11107,#8911,#8912);
#7278=AXIS2_PLACEMENT_3D('',#11109,#8913,#8914);
#7279=AXIS2_PLACEMENT_3D('',#11111,#8915,#8916);
#7280=AXIS2_PLACEMENT_3D('',#11113,#8917,#8918);
#7281=AXIS2_PLACEMENT_3D('',#11115,#8919,#8920);
#7282=AXIS2_PLACEMENT_3D('',#11116,#8921,#8922);
#7283=AXIS2_PLACEMENT_3D('',#11118,#8923,#8924);
#7284=AXIS2_PLACEMENT_3D('',#11120,#8925,#8926);
#7285=AXIS2_PLACEMENT_3D('',#11122,#8927,#8928);
#7286=AXIS2_PLACEMENT_3D('',#11124,#8929,#8930);
#7287=AXIS2_PLACEMENT_3D('',#11125,#8931,#8932);
#7288=AXIS2_PLACEMENT_3D('',#11127,#8933,#8934);
#7289=AXIS2_PLACEMENT_3D('',#11129,#8935,#8936);
#7290=AXIS2_PLACEMENT_3D('',#11131,#8937,#8938);
#7291=AXIS2_PLACEMENT_3D('',#11133,#8939,#8940);
#7292=AXIS2_PLACEMENT_3D('',#11134,#8941,#8942);
#7293=AXIS2_PLACEMENT_3D('',#11136,#8943,#8944);
#7294=AXIS2_PLACEMENT_3D('',#11138,#8945,#8946);
#7295=AXIS2_PLACEMENT_3D('',#11140,#8947,#8948);
#7296=AXIS2_PLACEMENT_3D('',#11142,#8949,#8950);
#7297=AXIS2_PLACEMENT_3D('',#11143,#8951,#8952);
#7298=AXIS2_PLACEMENT_3D('',#11145,#8953,#8954);
#7299=AXIS2_PLACEMENT_3D('',#11147,#8955,#8956);
#7300=AXIS2_PLACEMENT_3D('',#11149,#8957,#8958);
#7301=AXIS2_PLACEMENT_3D('',#11151,#8959,#8960);
#7302=AXIS2_PLACEMENT_3D('',#11152,#8961,#8962);
#7303=AXIS2_PLACEMENT_3D('',#11154,#8963,#8964);
#7304=AXIS2_PLACEMENT_3D('',#11156,#8965,#8966);
#7305=AXIS2_PLACEMENT_3D('',#11158,#8967,#8968);
#7306=AXIS2_PLACEMENT_3D('',#11160,#8969,#8970);
#7307=AXIS2_PLACEMENT_3D('',#11161,#8971,#8972);
#7308=AXIS2_PLACEMENT_3D('',#11163,#8973,#8974);
#7309=AXIS2_PLACEMENT_3D('',#11165,#8975,#8976);
#7310=AXIS2_PLACEMENT_3D('',#11167,#8977,#8978);
#7311=AXIS2_PLACEMENT_3D('',#11168,#8979,#8980);
#7312=AXIS2_PLACEMENT_3D('',#11174,#8984,#8985);
#7313=AXIS2_PLACEMENT_3D('',#11176,#8987,#8988);
#7314=AXIS2_PLACEMENT_3D('',#11178,#8990,#8991);
#7315=AXIS2_PLACEMENT_3D('',#11180,#8993,#8994);
#7316=AXIS2_PLACEMENT_3D('',#11183,#8997,#8998);
#7317=AXIS2_PLACEMENT_3D('',#11184,#8999,#9000);
#7318=AXIS2_PLACEMENT_3D('',#11185,#9001,#9002);
#7319=AXIS2_PLACEMENT_3D('',#11187,#9004,#9005);
#7320=AXIS2_PLACEMENT_3D('',#11189,#9007,#9008);
#7321=AXIS2_PLACEMENT_3D('',#11191,#9010,#9011);
#7322=AXIS2_PLACEMENT_3D('',#11193,#9013,#9014);
#7323=AXIS2_PLACEMENT_3D('',#11194,#9015,#9016);
#7324=AXIS2_PLACEMENT_3D('',#11195,#9017,#9018);
#7325=AXIS2_PLACEMENT_3D('',#11197,#9020,#9021);
#7326=AXIS2_PLACEMENT_3D('',#11199,#9023,#9024);
#7327=AXIS2_PLACEMENT_3D('',#11200,#9025,#9026);
#7328=AXIS2_PLACEMENT_3D('',#11201,#9027,#9028);
#7329=AXIS2_PLACEMENT_3D('',#11203,#9030,#9031);
#7330=AXIS2_PLACEMENT_3D('',#11205,#9033,#9034);
#7331=AXIS2_PLACEMENT_3D('',#11206,#9035,#9036);
#7332=AXIS2_PLACEMENT_3D('',#11207,#9037,#9038);
#7333=AXIS2_PLACEMENT_3D('',#11209,#9040,#9041);
#7334=AXIS2_PLACEMENT_3D('',#11211,#9043,#9044);
#7335=AXIS2_PLACEMENT_3D('',#11212,#9045,#9046);
#7336=AXIS2_PLACEMENT_3D('',#11213,#9047,#9048);
#7337=AXIS2_PLACEMENT_3D('',#11215,#9050,#9051);
#7338=AXIS2_PLACEMENT_3D('',#11217,#9053,#9054);
#7339=AXIS2_PLACEMENT_3D('',#11218,#9055,#9056);
#7340=AXIS2_PLACEMENT_3D('',#11219,#9057,#9058);
#7341=AXIS2_PLACEMENT_3D('',#11221,#9060,#9061);
#7342=AXIS2_PLACEMENT_3D('',#11223,#9063,#9064);
#7343=AXIS2_PLACEMENT_3D('',#11224,#9065,#9066);
#7344=AXIS2_PLACEMENT_3D('',#11226,#9068,#9069);
#7345=AXIS2_PLACEMENT_3D('',#11227,#9070,#9071);
#7346=AXIS2_PLACEMENT_3D('',#11229,#9073,#9074);
#7347=AXIS2_PLACEMENT_3D('',#11230,#9075,#9076);
#7348=AXIS2_PLACEMENT_3D('',#11232,#9078,#9079);
#7349=AXIS2_PLACEMENT_3D('',#11233,#9080,#9081);
#7350=AXIS2_PLACEMENT_3D('',#11235,#9083,#9084);
#7351=AXIS2_PLACEMENT_3D('',#11236,#9085,#9086);
#7352=AXIS2_PLACEMENT_3D('',#11238,#9088,#9089);
#7353=AXIS2_PLACEMENT_3D('',#11239,#9090,#9091);
#7354=AXIS2_PLACEMENT_3D('',#11241,#9093,#9094);
#7355=AXIS2_PLACEMENT_3D('',#11242,#9095,#9096);
#7356=AXIS2_PLACEMENT_3D('',#11244,#9098,#9099);
#7357=AXIS2_PLACEMENT_3D('',#11245,#9100,#9101);
#7358=AXIS2_PLACEMENT_3D('',#11247,#9103,#9104);
#7359=AXIS2_PLACEMENT_3D('',#11248,#9105,#9106);
#7360=AXIS2_PLACEMENT_3D('',#11250,#9108,#9109);
#7361=AXIS2_PLACEMENT_3D('',#11251,#9110,#9111);
#7362=AXIS2_PLACEMENT_3D('',#11253,#9113,#9114);
#7363=AXIS2_PLACEMENT_3D('',#11254,#9115,#9116);
#7364=AXIS2_PLACEMENT_3D('',#11256,#9118,#9119);
#7365=AXIS2_PLACEMENT_3D('',#11258,#9121,#9122);
#7366=AXIS2_PLACEMENT_3D('',#11259,#9123,#9124);
#7367=AXIS2_PLACEMENT_3D('',#11261,#9126,#9127);
#7368=AXIS2_PLACEMENT_3D('',#11263,#9129,#9130);
#7369=AXIS2_PLACEMENT_3D('',#11264,#9131,#9132);
#7370=AXIS2_PLACEMENT_3D('',#11266,#9134,#9135);
#7371=AXIS2_PLACEMENT_3D('',#11268,#9137,#9138);
#7372=AXIS2_PLACEMENT_3D('',#11269,#9139,#9140);
#7373=AXIS2_PLACEMENT_3D('',#11271,#9142,#9143);
#7374=AXIS2_PLACEMENT_3D('',#11273,#9145,#9146);
#7375=AXIS2_PLACEMENT_3D('',#11274,#9147,#9148);
#7376=AXIS2_PLACEMENT_3D('',#11276,#9150,#9151);
#7377=AXIS2_PLACEMENT_3D('',#11278,#9153,#9154);
#7378=AXIS2_PLACEMENT_3D('',#11280,#9156,#9157);
#7379=AXIS2_PLACEMENT_3D('',#11282,#9159,#9160);
#7380=AXIS2_PLACEMENT_3D('',#11283,#9161,#9162);
#7381=AXIS2_PLACEMENT_3D('',#11285,#9164,#9165);
#7382=AXIS2_PLACEMENT_3D('',#11287,#9167,#9168);
#7383=AXIS2_PLACEMENT_3D('',#11289,#9170,#9171);
#7384=AXIS2_PLACEMENT_3D('',#11291,#9173,#9174);
#7385=AXIS2_PLACEMENT_3D('',#11292,#9175,#9176);
#7386=AXIS2_PLACEMENT_3D('',#11294,#9178,#9179);
#7387=AXIS2_PLACEMENT_3D('',#11296,#9181,#9182);
#7388=AXIS2_PLACEMENT_3D('',#11298,#9184,#9185);
#7389=AXIS2_PLACEMENT_3D('',#11300,#9187,#9188);
#7390=AXIS2_PLACEMENT_3D('',#11301,#9189,#9190);
#7391=AXIS2_PLACEMENT_3D('',#11303,#9192,#9193);
#7392=AXIS2_PLACEMENT_3D('',#11305,#9195,#9196);
#7393=AXIS2_PLACEMENT_3D('',#11307,#9198,#9199);
#7394=AXIS2_PLACEMENT_3D('',#11309,#9201,#9202);
#7395=AXIS2_PLACEMENT_3D('',#11310,#9203,#9204);
#7396=AXIS2_PLACEMENT_3D('',#11312,#9206,#9207);
#7397=AXIS2_PLACEMENT_3D('',#11314,#9209,#9210);
#7398=AXIS2_PLACEMENT_3D('',#11316,#9212,#9213);
#7399=AXIS2_PLACEMENT_3D('',#11318,#9215,#9216);
#7400=AXIS2_PLACEMENT_3D('',#11319,#9217,#9218);
#7401=AXIS2_PLACEMENT_3D('',#11321,#9220,#9221);
#7402=AXIS2_PLACEMENT_3D('',#11323,#9223,#9224);
#7403=AXIS2_PLACEMENT_3D('',#11325,#9226,#9227);
#7404=AXIS2_PLACEMENT_3D('',#11327,#9229,#9230);
#7405=AXIS2_PLACEMENT_3D('',#11328,#9231,#9232);
#7406=AXIS2_PLACEMENT_3D('',#11330,#9234,#9235);
#7407=AXIS2_PLACEMENT_3D('',#11332,#9237,#9238);
#7408=AXIS2_PLACEMENT_3D('',#11334,#9240,#9241);
#7409=AXIS2_PLACEMENT_3D('',#11336,#9243,#9244);
#7410=AXIS2_PLACEMENT_3D('',#11337,#9245,#9246);
#7411=AXIS2_PLACEMENT_3D('',#11339,#9248,#9249);
#7412=AXIS2_PLACEMENT_3D('',#11341,#9251,#9252);
#7413=AXIS2_PLACEMENT_3D('',#11343,#9254,#9255);
#7414=AXIS2_PLACEMENT_3D('',#11345,#9257,#9258);
#7415=AXIS2_PLACEMENT_3D('',#11346,#9259,#9260);
#7416=AXIS2_PLACEMENT_3D('',#11348,#9262,#9263);
#7417=AXIS2_PLACEMENT_3D('',#11350,#9265,#9266);
#7418=AXIS2_PLACEMENT_3D('',#11352,#9268,#9269);
#7419=AXIS2_PLACEMENT_3D('',#11354,#9271,#9272);
#7420=AXIS2_PLACEMENT_3D('',#11355,#9273,#9274);
#7421=AXIS2_PLACEMENT_3D('',#11357,#9276,#9277);
#7422=AXIS2_PLACEMENT_3D('',#11359,#9279,#9280);
#7423=AXIS2_PLACEMENT_3D('',#11361,#9282,#9283);
#7424=AXIS2_PLACEMENT_3D('',#11363,#9285,#9286);
#7425=AXIS2_PLACEMENT_3D('',#11364,#9287,#9288);
#7426=AXIS2_PLACEMENT_3D('',#11366,#9290,#9291);
#7427=AXIS2_PLACEMENT_3D('',#11368,#9293,#9294);
#7428=AXIS2_PLACEMENT_3D('',#11370,#9296,#9297);
#7429=AXIS2_PLACEMENT_3D('',#11372,#9299,#9300);
#7430=AXIS2_PLACEMENT_3D('',#11373,#9301,#9302);
#7431=AXIS2_PLACEMENT_3D('',#11375,#9304,#9305);
#7432=AXIS2_PLACEMENT_3D('',#11377,#9307,#9308);
#7433=AXIS2_PLACEMENT_3D('',#11379,#9310,#9311);
#7434=AXIS2_PLACEMENT_3D('',#11381,#9313,#9314);
#7435=AXIS2_PLACEMENT_3D('',#11382,#9315,#9316);
#7436=AXIS2_PLACEMENT_3D('',#11384,#9318,#9319);
#7437=AXIS2_PLACEMENT_3D('',#11386,#9321,#9322);
#7438=AXIS2_PLACEMENT_3D('',#11388,#9324,#9325);
#7439=AXIS2_PLACEMENT_3D('',#11390,#9327,#9328);
#7440=AXIS2_PLACEMENT_3D('',#11391,#9329,#9330);
#7441=AXIS2_PLACEMENT_3D('',#11393,#9332,#9333);
#7442=AXIS2_PLACEMENT_3D('',#11395,#9335,#9336);
#7443=AXIS2_PLACEMENT_3D('',#11397,#9338,#9339);
#7444=AXIS2_PLACEMENT_3D('',#11399,#9341,#9342);
#7445=AXIS2_PLACEMENT_3D('',#11400,#9343,#9344);
#7446=AXIS2_PLACEMENT_3D('',#11402,#9346,#9347);
#7447=AXIS2_PLACEMENT_3D('',#11404,#9349,#9350);
#8063=DIRECTION('axis',(0.,0.,1.));
#8064=DIRECTION('refdir',(1.,0.,0.));
#8065=DIRECTION('center_axis',(0.,0.,1.));
#8066=DIRECTION('ref_axis',(-1.83697019872103E-16,-1.,0.));
#8067=DIRECTION('center_axis',(0.,0.,1.));
#8068=DIRECTION('ref_axis',(1.,0.,0.));
#8069=DIRECTION('',(0.,0.,1.));
#8070=DIRECTION('center_axis',(0.,0.,1.));
#8071=DIRECTION('ref_axis',(1.,0.,0.));
#8072=DIRECTION('',(0.,0.,1.));
#8073=DIRECTION('center_axis',(0.,0.,-1.));
#8074=DIRECTION('ref_axis',(-1.,0.,0.));
#8075=DIRECTION('center_axis',(0.,0.,-1.));
#8076=DIRECTION('ref_axis',(-1.,0.,0.));
#8077=DIRECTION('',(0.,0.,1.));
#8078=DIRECTION('center_axis',(0.,0.,1.));
#8079=DIRECTION('ref_axis',(1.,0.,0.));
#8080=DIRECTION('',(0.,0.,-1.));
#8081=DIRECTION('center_axis',(0.,0.,1.));
#8082=DIRECTION('ref_axis',(1.,0.,0.));
#8083=DIRECTION('center_axis',(0.,0.,-1.));
#8084=DIRECTION('ref_axis',(-1.,0.,0.));
#8085=DIRECTION('',(0.,0.,-1.));
#8086=DIRECTION('center_axis',(0.,0.,-1.));
#8087=DIRECTION('ref_axis',(-1.,0.,0.));
#8088=DIRECTION('center_axis',(0.,0.,-1.));
#8089=DIRECTION('ref_axis',(-1.,0.,0.));
#8090=DIRECTION('center_axis',(0.,0.,-1.));
#8091=DIRECTION('ref_axis',(-1.,0.,0.));
#8092=DIRECTION('',(0.,0.,1.));
#8093=DIRECTION('center_axis',(0.,0.,1.));
#8094=DIRECTION('ref_axis',(1.,0.,0.));
#8095=DIRECTION('',(0.,0.,-1.));
#8096=DIRECTION('center_axis',(0.,0.,1.));
#8097=DIRECTION('ref_axis',(1.,0.,0.));
#8098=DIRECTION('center_axis',(0.,0.,-1.));
#8099=DIRECTION('ref_axis',(-1.,0.,0.));
#8100=DIRECTION('',(0.,0.,-1.));
#8101=DIRECTION('center_axis',(0.,0.,-1.));
#8102=DIRECTION('ref_axis',(-1.,0.,0.));
#8103=DIRECTION('center_axis',(0.,0.,-1.));
#8104=DIRECTION('ref_axis',(-1.,0.,0.));
#8105=DIRECTION('center_axis',(0.,0.,-1.));
#8106=DIRECTION('ref_axis',(-1.,0.,0.));
#8107=DIRECTION('',(0.,0.,1.));
#8108=DIRECTION('center_axis',(0.,0.,1.));
#8109=DIRECTION('ref_axis',(1.,0.,0.));
#8110=DIRECTION('',(0.,0.,-1.));
#8111=DIRECTION('center_axis',(0.,0.,1.));
#8112=DIRECTION('ref_axis',(1.,0.,0.));
#8113=DIRECTION('center_axis',(1.34209460732156E-15,-2.06113990643666E-16,
-1.));
#8114=DIRECTION('ref_axis',(-1.,2.14280619850583E-33,-1.34209460732156E-15));
#8115=DIRECTION('center_axis',(0.,0.,-1.));
#8116=DIRECTION('ref_axis',(-1.,0.,0.));
#8117=DIRECTION('',(0.,0.,1.));
#8118=DIRECTION('center_axis',(0.,0.,-1.));
#8119=DIRECTION('ref_axis',(-1.,0.,0.));
#8120=DIRECTION('center_axis',(0.,0.,-1.));
#8121=DIRECTION('ref_axis',(-1.,0.,0.));
#8122=DIRECTION('',(0.,0.,1.));
#8123=DIRECTION('center_axis',(0.,0.,1.));
#8124=DIRECTION('ref_axis',(1.,0.,0.));
#8125=DIRECTION('',(0.,0.,-1.));
#8126=DIRECTION('center_axis',(0.,0.,1.));
#8127=DIRECTION('ref_axis',(1.,0.,0.));
#8128=DIRECTION('center_axis',(0.,0.,-1.));
#8129=DIRECTION('ref_axis',(-1.,0.,0.));
#8130=DIRECTION('center_axis',(-1.3556201284053E-15,-7.74272536198527E-17,
-1.));
#8131=DIRECTION('ref_axis',(-1.,2.42293261278703E-34,1.3556201284053E-15));
#8132=DIRECTION('',(0.,0.,1.));
#8133=DIRECTION('center_axis',(0.,0.,-1.));
#8134=DIRECTION('ref_axis',(-1.,0.,0.));
#8135=DIRECTION('center_axis',(0.,0.,-1.));
#8136=DIRECTION('ref_axis',(-1.,0.,0.));
#8137=DIRECTION('',(0.,0.,1.));
#8138=DIRECTION('center_axis',(0.,0.,1.));
#8139=DIRECTION('ref_axis',(1.,0.,0.));
#8140=DIRECTION('',(0.,0.,-1.));
#8141=DIRECTION('center_axis',(0.,0.,-1.));
#8142=DIRECTION('ref_axis',(-1.,0.,0.));
#8143=DIRECTION('center_axis',(0.,0.,-1.));
#8144=DIRECTION('ref_axis',(-1.,0.,0.));
#8145=DIRECTION('',(0.,0.,1.));
#8146=DIRECTION('center_axis',(0.,0.,1.));
#8147=DIRECTION('ref_axis',(1.,0.,0.));
#8148=DIRECTION('',(0.,0.,-1.));
#8149=DIRECTION('center_axis',(0.,0.,-1.));
#8150=DIRECTION('ref_axis',(-1.,0.,0.));
#8151=DIRECTION('center_axis',(-2.13696732994728E-15,-4.30864304074819E-16,
-1.));
#8152=DIRECTION('ref_axis',(-1.,-1.17354868605786E-31,2.13696732994728E-15));
#8153=DIRECTION('',(0.,0.,1.));
#8154=DIRECTION('center_axis',(-2.13696732994728E-15,-4.30864304074819E-16,
1.));
#8155=DIRECTION('ref_axis',(1.,1.17354868605786E-31,2.13696732994728E-15));
#8156=DIRECTION('',(0.,0.,-1.));
#8157=DIRECTION('center_axis',(0.,0.,-1.));
#8158=DIRECTION('ref_axis',(-1.,0.,0.));
#8159=DIRECTION('center_axis',(0.,0.,-1.));
#8160=DIRECTION('ref_axis',(-1.,0.,0.));
#8161=DIRECTION('',(0.,0.,1.));
#8162=DIRECTION('center_axis',(0.,0.,1.));
#8163=DIRECTION('ref_axis',(1.,0.,0.));
#8164=DIRECTION('',(0.,0.,-1.));
#8165=DIRECTION('center_axis',(0.,0.,-1.));
#8166=DIRECTION('ref_axis',(-1.,0.,0.));
#8167=DIRECTION('center_axis',(1.77696849674338E-15,1.26279704599331E-15,
-1.));
#8168=DIRECTION('ref_axis',(-1.,2.15613826771123E-31,-1.77696849674338E-15));
#8169=DIRECTION('',(0.,0.,1.));
#8170=DIRECTION('center_axis',(1.77696849674338E-15,1.26279704599331E-15,
1.));
#8171=DIRECTION('ref_axis',(1.,-2.15613826771123E-31,-1.77696849674338E-15));
#8172=DIRECTION('',(0.,0.,-1.));
#8173=DIRECTION('center_axis',(0.,0.,-1.));
#8174=DIRECTION('ref_axis',(-1.,0.,0.));
#8175=DIRECTION('center_axis',(0.,0.,-1.));
#8176=DIRECTION('ref_axis',(-1.,0.,0.));
#8177=DIRECTION('',(0.,0.,1.));
#8178=DIRECTION('center_axis',(0.,0.,1.));
#8179=DIRECTION('ref_axis',(1.,0.,0.));
#8180=DIRECTION('',(0.,0.,-1.));
#8181=DIRECTION('center_axis',(0.,0.,-1.));
#8182=DIRECTION('ref_axis',(-1.,0.,0.));
#8183=DIRECTION('center_axis',(0.,0.,-1.));
#8184=DIRECTION('ref_axis',(-1.,0.,0.));
#8185=DIRECTION('',(0.,0.,1.));
#8186=DIRECTION('center_axis',(0.,0.,1.));
#8187=DIRECTION('ref_axis',(1.,0.,0.));
#8188=DIRECTION('',(0.,0.,-1.));
#8189=DIRECTION('center_axis',(0.,0.,-1.));
#8190=DIRECTION('ref_axis',(-1.,0.,0.));
#8191=DIRECTION('center_axis',(0.,0.,-1.));
#8192=DIRECTION('ref_axis',(-1.,0.,0.));
#8193=DIRECTION('',(0.,0.,1.));
#8194=DIRECTION('center_axis',(0.,0.,1.));
#8195=DIRECTION('ref_axis',(1.,0.,0.));
#8196=DIRECTION('',(0.,0.,-1.));
#8197=DIRECTION('center_axis',(0.,0.,-1.));
#8198=DIRECTION('ref_axis',(-1.,0.,0.));
#8199=DIRECTION('center_axis',(-2.13696732994721E-15,4.30864304074825E-16,
-1.));
#8200=DIRECTION('ref_axis',(-1.,1.17354868605837E-31,2.13696732994721E-15));
#8201=DIRECTION('',(0.,0.,1.));
#8202=DIRECTION('center_axis',(-2.13696732994721E-15,4.30864304074825E-16,
1.));
#8203=DIRECTION('ref_axis',(1.,-1.17354868605837E-31,2.13696732994721E-15));
#8204=DIRECTION('',(0.,0.,-1.));
#8205=DIRECTION('center_axis',(0.,0.,-1.));
#8206=DIRECTION('ref_axis',(-1.,0.,0.));
#8207=DIRECTION('center_axis',(0.,0.,-1.));
#8208=DIRECTION('ref_axis',(-1.,0.,0.));
#8209=DIRECTION('',(0.,0.,1.));
#8210=DIRECTION('center_axis',(0.,0.,1.));
#8211=DIRECTION('ref_axis',(1.,0.,0.));
#8212=DIRECTION('',(0.,0.,-1.));
#8213=DIRECTION('center_axis',(0.,0.,-1.));
#8214=DIRECTION('ref_axis',(-1.,0.,0.));
#8215=DIRECTION('center_axis',(-3.9743489494276E-14,0.,1.));
#8216=DIRECTION('ref_axis',(1.,0.,3.9743489494276E-14));
#8217=DIRECTION('',(0.,0.,-1.));
#8218=DIRECTION('center_axis',(3.9743489494276E-14,0.,1.));
#8219=DIRECTION('ref_axis',(1.,0.,-3.9743489494276E-14));
#8220=DIRECTION('',(0.,0.,1.));
#8221=DIRECTION('center_axis',(0.,0.,-1.));
#8222=DIRECTION('ref_axis',(-1.,0.,0.));
#8223=DIRECTION('center_axis',(-2.65935852241228E-14,-2.95351685640873E-14,
1.));
#8224=DIRECTION('ref_axis',(1.52054869890062E-31,-1.,-2.95351685640873E-14));
#8225=DIRECTION('',(0.,0.,-1.));
#8226=DIRECTION('center_axis',(2.65935852241255E-14,2.95351685640904E-14,
1.));
#8227=DIRECTION('ref_axis',(1.52054870042792E-31,-1.,2.95351685640904E-14));
#8228=DIRECTION('',(0.,0.,1.));
#8229=DIRECTION('center_axis',(0.,0.,-1.));
#8230=DIRECTION('ref_axis',(-1.,0.,0.));
#8231=DIRECTION('center_axis',(3.21531584166429E-14,2.33606369993845E-14,
1.));
#8232=DIRECTION('ref_axis',(1.,-8.29846859020713E-32,-3.21531584166429E-14));
#8233=DIRECTION('',(0.,0.,1.));
#8234=DIRECTION('center_axis',(-3.21531584166387E-14,-2.33606369993815E-14,
1.));
#8235=DIRECTION('ref_axis',(1.,-8.29846856946285E-32,3.21531584166387E-14));
#8236=DIRECTION('',(0.,0.,-1.));
#8237=DIRECTION('center_axis',(0.,0.,-1.));
#8238=DIRECTION('ref_axis',(-1.,0.,0.));
#8239=DIRECTION('center_axis',(-1.98717447471412E-14,-3.44188715370884E-14,
1.));
#8240=DIRECTION('ref_axis',(-9.03655535160673E-32,-1.,-3.44188715370884E-14));
#8241=DIRECTION('',(0.,0.,-1.));
#8242=DIRECTION('center_axis',(1.98717447471412E-14,3.44188715370884E-14,
1.));
#8243=DIRECTION('ref_axis',(-9.03655535160673E-32,-1.,3.44188715370884E-14));
#8244=DIRECTION('',(0.,0.,1.));
#8245=DIRECTION('center_axis',(0.,0.,-1.));
#8246=DIRECTION('ref_axis',(-1.,0.,0.));
#8247=DIRECTION('center_axis',(-1.22814136694924E-14,-3.77983046638355E-14,
1.));
#8248=DIRECTION('ref_axis',(2.22571381162951E-32,-1.,-3.77983046638355E-14));
#8249=DIRECTION('',(0.,0.,-1.));
#8250=DIRECTION('center_axis',(1.22814136694963E-14,3.7798304663847E-14,
1.));
#8251=DIRECTION('ref_axis',(2.22571383838198E-32,-1.,3.7798304663847E-14));
#8252=DIRECTION('',(0.,0.,1.));
#8253=DIRECTION('center_axis',(0.,0.,-1.));
#8254=DIRECTION('ref_axis',(-1.,0.,0.));
#8255=DIRECTION('center_axis',(3.63074842983588E-14,1.61651335010186E-14,
1.));
#8256=DIRECTION('ref_axis',(1.,-2.86104045702539E-32,-3.63074842983588E-14));
#8257=DIRECTION('',(0.,0.,1.));
#8258=DIRECTION('center_axis',(-3.63074842983588E-14,-1.61651335010186E-14,
1.));
#8259=DIRECTION('ref_axis',(1.,-2.86104045702539E-32,3.63074842983588E-14));
#8260=DIRECTION('',(0.,0.,-1.));
#8261=DIRECTION('center_axis',(0.,0.,-1.));
#8262=DIRECTION('ref_axis',(-1.,0.,0.));
#8263=DIRECTION('center_axis',(3.88749988936205E-14,8.263136099754E-15,
1.));
#8264=DIRECTION('ref_axis',(1.,4.7064185543995E-32,-3.88749988936205E-14));
#8265=DIRECTION('',(0.,0.,1.));
#8266=DIRECTION('center_axis',(-3.88749988936141E-14,-8.26313609975264E-15,
1.));
#8267=DIRECTION('ref_axis',(1.,4.70641856382513E-32,3.88749988936141E-14));
#8268=DIRECTION('',(0.,0.,-1.));
#8269=DIRECTION('center_axis',(0.,0.,-1.));
#8270=DIRECTION('ref_axis',(-1.,0.,0.));
#8271=DIRECTION('center_axis',(3.88749988936198E-14,-8.26313609975388E-15,
1.));
#8272=DIRECTION('ref_axis',(1.,-4.70641855550782E-32,-3.88749988936198E-14));
#8273=DIRECTION('',(0.,0.,1.));
#8274=DIRECTION('center_axis',(-3.88749988936198E-14,8.2631360997538E-15,
1.));
#8275=DIRECTION('ref_axis',(1.,-4.70641855495463E-32,3.88749988936198E-14));
#8276=DIRECTION('',(0.,0.,-1.));
#8277=DIRECTION('center_axis',(0.,0.,-1.));
#8278=DIRECTION('ref_axis',(-1.,0.,0.));
#8279=DIRECTION('center_axis',(-1.98717447471421E-14,3.44188715370906E-14,
1.));
#8280=DIRECTION('ref_axis',(9.03655534251286E-32,-1.,3.44188715370906E-14));
#8281=DIRECTION('',(0.,0.,-1.));
#8282=DIRECTION('center_axis',(1.98717447471421E-14,-3.44188715370906E-14,
1.));
#8283=DIRECTION('ref_axis',(9.03655534251286E-32,-1.,-3.44188715370906E-14));
#8284=DIRECTION('',(0.,0.,1.));
#8285=DIRECTION('center_axis',(0.,0.,-1.));
#8286=DIRECTION('ref_axis',(-1.,0.,0.));
#8287=DIRECTION('center_axis',(-2.65935852241256E-14,2.95351685640909E-14,
1.));
#8288=DIRECTION('ref_axis',(-1.52054870064765E-31,-1.,2.95351685640909E-14));
#8289=DIRECTION('',(0.,0.,-1.));
#8290=DIRECTION('center_axis',(2.65935852241255E-14,-2.95351685640905E-14,
1.));
#8291=DIRECTION('ref_axis',(-1.52054870032748E-31,-1.,-2.95351685640905E-14));
#8292=DIRECTION('',(0.,0.,1.));
#8293=DIRECTION('center_axis',(0.,0.,-1.));
#8294=DIRECTION('ref_axis',(-1.,0.,0.));
#8295=DIRECTION('center_axis',(3.6307484298364E-14,-1.61651335010211E-14,
1.));
#8296=DIRECTION('ref_axis',(1.,2.86104047421028E-32,-3.6307484298364E-14));
#8297=DIRECTION('',(0.,0.,1.));
#8298=DIRECTION('center_axis',(-3.6307484298364E-14,1.61651335010213E-14,
1.));
#8299=DIRECTION('ref_axis',(1.,2.86104047531475E-32,3.6307484298364E-14));
#8300=DIRECTION('',(0.,0.,-1.));
#8301=DIRECTION('center_axis',(0.,0.,-1.));
#8302=DIRECTION('ref_axis',(-1.,0.,0.));
#8303=DIRECTION('center_axis',(3.21531584166325E-14,-2.33606369993773E-14,
1.));
#8304=DIRECTION('ref_axis',(1.,8.29846854034834E-32,-3.21531584166325E-14));
#8305=DIRECTION('',(0.,0.,1.));
#8306=DIRECTION('center_axis',(-3.21531584166325E-14,2.33606369993773E-14,
1.));
#8307=DIRECTION('ref_axis',(1.,8.29846854034834E-32,3.21531584166325E-14));
#8308=DIRECTION('',(0.,0.,-1.));
#8309=DIRECTION('center_axis',(0.,0.,-1.));
#8310=DIRECTION('ref_axis',(-1.,0.,0.));
#8311=DIRECTION('center_axis',(1.22814136694964E-14,-3.77983046638479E-14,
1.));
#8312=DIRECTION('ref_axis',(-2.22571383991556E-32,-1.,-3.77983046638479E-14));
#8313=DIRECTION('',(0.,0.,1.));
#8314=DIRECTION('center_axis',(-1.2281413669496E-14,3.7798304663847E-14,
1.));
#8315=DIRECTION('ref_axis',(-2.22571383826539E-32,-1.,3.7798304663847E-14));
#8316=DIRECTION('',(0.,0.,-1.));
#8317=DIRECTION('center_axis',(0.,0.,-1.));
#8318=DIRECTION('ref_axis',(-1.,0.,0.));
#8319=DIRECTION('center_axis',(4.15432588173347E-15,-3.95257705004224E-14,
1.));
#8320=DIRECTION('ref_axis',(1.01104027071865E-32,-1.,-3.95257705004224E-14));
#8321=DIRECTION('',(0.,0.,1.));
#8322=DIRECTION('center_axis',(-4.15432588173344E-15,3.95257705004224E-14,
1.));
#8323=DIRECTION('ref_axis',(1.01104027037785E-32,-1.,3.95257705004224E-14));
#8324=DIRECTION('',(0.,0.,-1.));
#8325=DIRECTION('center_axis',(0.,0.,-1.));
#8326=DIRECTION('ref_axis',(-1.,0.,0.));
#8327=DIRECTION('center_axis',(-4.15432588173031E-15,-3.95257705003908E-14,
1.));
#8328=DIRECTION('ref_axis',(-1.01104028749611E-32,-1.,-3.95257705003908E-14));
#8329=DIRECTION('',(0.,0.,1.));
#8330=DIRECTION('center_axis',(4.1543258817303E-15,3.95257705003909E-14,
1.));
#8331=DIRECTION('ref_axis',(-1.0110402872876E-32,-1.,3.95257705003909E-14));
#8332=DIRECTION('center_axis',(0.,0.,-1.));
#8333=DIRECTION('ref_axis',(-1.,0.,0.));
#8334=DIRECTION('center_axis',(-1.22814136694946E-14,-3.77983046638411E-14,
1.));
#8335=DIRECTION('ref_axis',(2.22571382356633E-32,-1.,-3.77983046638411E-14));
#8336=DIRECTION('',(0.,0.,1.));
#8337=DIRECTION('center_axis',(1.22814136694949E-14,3.77983046638421E-14,
1.));
#8338=DIRECTION('ref_axis',(2.2257138263465E-32,-1.,3.77983046638421E-14));
#8339=DIRECTION('center_axis',(0.,0.,-1.));
#8340=DIRECTION('ref_axis',(-1.,0.,0.));
#8341=DIRECTION('center_axis',(1.22814136694957E-14,-3.77983046638471E-14,
1.));
#8342=DIRECTION('ref_axis',(-2.22571383862412E-32,-1.,-3.77983046638471E-14));
#8343=DIRECTION('',(0.,0.,-1.));
#8344=DIRECTION('center_axis',(-1.22814136694957E-14,3.77983046638471E-14,
1.));
#8345=DIRECTION('ref_axis',(-2.22571383862412E-32,-1.,3.77983046638471E-14));
#8346=DIRECTION('center_axis',(0.,0.,-1.));
#8347=DIRECTION('ref_axis',(-1.,0.,0.));
#8348=DIRECTION('center_axis',(1.9871744747142E-14,-3.44188715370905E-14,
1.));
#8349=DIRECTION('ref_axis',(9.03655534124833E-32,-1.,-3.44188715370905E-14));
#8350=DIRECTION('',(0.,0.,-1.));
#8351=DIRECTION('center_axis',(-1.98717447471409E-14,3.44188715370886E-14,
1.));
#8352=DIRECTION('ref_axis',(9.03655535174126E-32,-1.,3.44188715370886E-14));
#8353=DIRECTION('',(0.,0.,1.));
#8354=DIRECTION('center_axis',(0.,0.,-1.));
#8355=DIRECTION('ref_axis',(-1.,0.,0.));
#8356=DIRECTION('center_axis',(3.21531584166354E-14,-2.33606369993796E-14,
1.));
#8357=DIRECTION('ref_axis',(1.,8.29846855706183E-32,-3.21531584166354E-14));
#8358=DIRECTION('',(0.,0.,-1.));
#8359=DIRECTION('center_axis',(-3.21531584166371E-14,2.33606369993811E-14,
1.));
#8360=DIRECTION('ref_axis',(1.,8.29846856272883E-32,3.21531584166371E-14));
#8361=DIRECTION('',(0.,0.,1.));
#8362=DIRECTION('center_axis',(0.,0.,-1.));
#8363=DIRECTION('ref_axis',(-1.,0.,0.));
#8364=DIRECTION('center_axis',(-2.65935852241255E-14,2.9535168564091E-14,
1.));
#8365=DIRECTION('ref_axis',(-1.52054870065482E-31,-1.,2.9535168564091E-14));
#8366=DIRECTION('',(0.,0.,1.));
#8367=DIRECTION('center_axis',(2.65935852241255E-14,-2.9535168564091E-14,
1.));
#8368=DIRECTION('ref_axis',(-1.52054870065482E-31,-1.,-2.9535168564091E-14));
#8369=DIRECTION('',(0.,0.,-1.));
#8370=DIRECTION('center_axis',(0.,0.,-1.));
#8371=DIRECTION('ref_axis',(-1.,0.,0.));
#8372=DIRECTION('center_axis',(3.6307484298364E-14,-1.61651335010214E-14,
1.));
#8373=DIRECTION('ref_axis',(1.,2.86104047630569E-32,-3.6307484298364E-14));
#8374=DIRECTION('',(0.,0.,-1.));
#8375=DIRECTION('center_axis',(-3.6307484298364E-14,1.61651335010214E-14,
1.));
#8376=DIRECTION('ref_axis',(1.,2.86104047630569E-32,3.6307484298364E-14));
#8377=DIRECTION('',(0.,0.,1.));
#8378=DIRECTION('center_axis',(0.,0.,-1.));
#8379=DIRECTION('ref_axis',(-1.,0.,0.));
#8380=DIRECTION('center_axis',(3.8874998893626E-14,-8.26313609975566E-15,
1.));
#8381=DIRECTION('ref_axis',(1.,-4.7064185451803E-32,-3.8874998893626E-14));
#8382=DIRECTION('',(0.,0.,-1.));
#8383=DIRECTION('center_axis',(-3.8874998893626E-14,8.26313609975566E-15,
1.));
#8384=DIRECTION('ref_axis',(1.,-4.7064185451803E-32,3.8874998893626E-14));
#8385=DIRECTION('',(0.,0.,1.));
#8386=DIRECTION('center_axis',(0.,0.,-1.));
#8387=DIRECTION('ref_axis',(1.,-1.00915871466367E-14,0.));
#8388=DIRECTION('center_axis',(3.9743489494276E-14,-6.0250801316063E-28,
1.));
#8389=DIRECTION('ref_axis',(1.,2.69212629025427E-45,-3.9743489494276E-14));
#8390=DIRECTION('',(0.,0.,-1.));
#8391=DIRECTION('center_axis',(-3.9743489494276E-14,6.0250801316063E-28,
1.));
#8392=DIRECTION('ref_axis',(1.,2.69212629025427E-45,3.9743489494276E-14));
#8393=DIRECTION('',(0.,0.,1.));
#8394=DIRECTION('center_axis',(0.,0.,-1.));
#8395=DIRECTION('ref_axis',(-1.,0.,0.));
#8396=DIRECTION('center_axis',(3.88749988936263E-14,8.26313609975447E-15,
1.));
#8397=DIRECTION('ref_axis',(1.,4.70641854477592E-32,-3.88749988936263E-14));
#8398=DIRECTION('',(0.,0.,-1.));
#8399=DIRECTION('center_axis',(-3.88749988936202E-14,-8.26313609975338E-15,
1.));
#8400=DIRECTION('ref_axis',(1.,4.70641855525022E-32,3.88749988936202E-14));
#8401=DIRECTION('',(0.,0.,1.));
#8402=DIRECTION('center_axis',(0.,0.,-1.));
#8403=DIRECTION('ref_axis',(-1.,0.,0.));
#8404=DIRECTION('center_axis',(2.65935852241261E-14,2.95351685640905E-14,
1.));
#8405=DIRECTION('ref_axis',(1.52054870048981E-31,-1.,2.95351685640905E-14));
#8406=DIRECTION('',(0.,0.,-1.));
#8407=DIRECTION('center_axis',(-2.65935852241231E-14,-2.9535168564087E-14,
1.));
#8408=DIRECTION('ref_axis',(1.52054869867193E-31,-1.,-2.9535168564087E-14));
#8409=DIRECTION('',(0.,0.,1.));
#8410=DIRECTION('center_axis',(0.,0.,-1.));
#8411=DIRECTION('ref_axis',(-1.,0.,0.));
#8412=DIRECTION('center_axis',(-1.98717447471434E-14,-3.44188715370916E-14,
1.));
#8413=DIRECTION('ref_axis',(-9.03655533788522E-32,-1.,-3.44188715370916E-14));
#8414=DIRECTION('',(0.,0.,1.));
#8415=DIRECTION('center_axis',(1.98717447471426E-14,3.44188715370902E-14,
1.));
#8416=DIRECTION('ref_axis',(-9.03655534129317E-32,-1.,3.44188715370902E-14));
#8417=DIRECTION('',(0.,0.,-1.));
#8418=DIRECTION('center_axis',(0.,0.,-1.));
#8419=DIRECTION('ref_axis',(-1.,0.,0.));
#8420=DIRECTION('center_axis',(-3.21531584166418E-14,-2.33606369993834E-14,
1.));
#8421=DIRECTION('ref_axis',(1.,-8.29846858379378E-32,3.21531584166418E-14));
#8422=DIRECTION('',(0.,0.,1.));
#8423=DIRECTION('center_axis',(3.21531584166388E-14,2.33606369993814E-14,
1.));
#8424=DIRECTION('ref_axis',(1.,-8.2984685715573E-32,-3.21531584166388E-14));
#8425=DIRECTION('',(0.,0.,-1.));
#8426=DIRECTION('center_axis',(0.,0.,-1.));
#8427=DIRECTION('ref_axis',(-1.,0.,0.));
#8428=DIRECTION('center_axis',(-3.63074842983631E-14,-1.616513350102E-14,
1.));
#8429=DIRECTION('ref_axis',(1.,-2.86104047041744E-32,3.63074842983631E-14));
#8430=DIRECTION('',(0.,0.,1.));
#8431=DIRECTION('center_axis',(3.63074842983642E-14,1.61651335010208E-14,
1.));
#8432=DIRECTION('ref_axis',(1.,-2.86104047448254E-32,-3.63074842983642E-14));
#8433=DIRECTION('',(0.,0.,-1.));
#8434=DIRECTION('center_axis',(0.,0.,-1.));
#8435=DIRECTION('ref_axis',(-1.,0.,0.));
#8436=DIRECTION('center_axis',(-4.15432588173083E-15,-3.95257705003972E-14,
1.));
#8437=DIRECTION('ref_axis',(-1.01104028692887E-32,-1.,-3.95257705003972E-14));
#8438=DIRECTION('',(0.,0.,-1.));
#8439=DIRECTION('center_axis',(4.15432588173083E-15,3.95257705003972E-14,
1.));
#8440=DIRECTION('ref_axis',(-1.01104028692887E-32,-1.,3.95257705003972E-14));
#8441=DIRECTION('',(0.,0.,1.));
#8442=DIRECTION('center_axis',(0.,0.,1.));
#8443=DIRECTION('ref_axis',(1.,0.,0.));
#8444=DIRECTION('center_axis',(-1.20692810937362E-15,6.22113696155732E-16,
-1.));
#8445=DIRECTION('ref_axis',(-1.,1.73910758130641E-32,1.20692810937362E-15));
#8446=DIRECTION('center_axis',(2.17985119260763E-15,2.28516055189852E-17,
1.));
#8447=DIRECTION('ref_axis',(1.,5.24414567525364E-33,-2.17985119260763E-15));
#8448=DIRECTION('center_axis',(0.,0.,-1.));
#8449=DIRECTION('ref_axis',(-1.,0.,0.));
#8450=DIRECTION('center_axis',(0.,0.,1.));
#8451=DIRECTION('ref_axis',(1.,0.,0.));
#8452=DIRECTION('center_axis',(0.,0.,-1.));
#8453=DIRECTION('ref_axis',(-1.,0.,0.));
#8454=DIRECTION('center_axis',(0.,0.,-1.));
#8455=DIRECTION('ref_axis',(-1.,0.,0.));
#8456=DIRECTION('center_axis',(0.,0.,1.));
#8457=DIRECTION('ref_axis',(1.,0.,0.));
#8458=DIRECTION('center_axis',(0.,0.,-1.));
#8459=DIRECTION('ref_axis',(-1.,0.,0.));
#8460=DIRECTION('center_axis',(0.,0.,1.));
#8461=DIRECTION('ref_axis',(1.,0.,0.));
#8462=DIRECTION('center_axis',(2.18703987820093E-16,-1.34010054766509E-15,
-1.));
#8463=DIRECTION('ref_axis',(-2.70980336596394E-33,1.,-1.34010054766509E-15));
#8464=DIRECTION('center_axis',(0.,0.,-1.));
#8465=DIRECTION('ref_axis',(-1.,0.,0.));
#8466=DIRECTION('center_axis',(0.,0.,1.));
#8467=DIRECTION('ref_axis',(1.,0.,0.));
#8468=DIRECTION('center_axis',(0.,0.,-1.));
#8469=DIRECTION('ref_axis',(-1.,0.,0.));
#8470=DIRECTION('center_axis',(0.,0.,1.));
#8471=DIRECTION('ref_axis',(1.,0.,0.));
#8472=DIRECTION('center_axis',(-6.4697789773716E-17,-1.35628725133693E-15,
-1.));
#8473=DIRECTION('ref_axis',(-2.45620303515543E-34,1.,-1.35628725133693E-15));
#8474=DIRECTION('center_axis',(0.,0.,-1.));
#8475=DIRECTION('ref_axis',(-1.,0.,0.));
#8476=DIRECTION('center_axis',(1.77696849674338E-15,-1.26279704599333E-15,
1.));
#8477=DIRECTION('ref_axis',(1.,2.1561382677115E-31,-1.77696849674338E-15));
#8478=DIRECTION('center_axis',(0.,0.,-1.));
#8479=DIRECTION('ref_axis',(-1.,0.,0.));
#8480=DIRECTION('center_axis',(1.47558720267693E-15,1.6046544254399E-15,
1.));
#8481=DIRECTION('ref_axis',(-2.31817004142331E-33,-1.,1.6046544254399E-15));
#8482=DIRECTION('center_axis',(0.,0.,-1.));
#8483=DIRECTION('ref_axis',(-1.,0.,0.));
#8484=DIRECTION('center_axis',(0.,0.,-1.));
#8485=DIRECTION('ref_axis',(-1.,0.,0.));
#8486=DIRECTION('center_axis',(0.,0.,1.));
#8487=DIRECTION('ref_axis',(1.,0.,0.));
#8488=DIRECTION('center_axis',(0.,0.,-1.));
#8489=DIRECTION('ref_axis',(-1.,0.,0.));
#8490=DIRECTION('center_axis',(0.,0.,1.));
#8491=DIRECTION('ref_axis',(1.,0.,0.));
#8492=DIRECTION('center_axis',(-6.10756095622581E-16,-1.21271509589043E-15,
-1.));
#8493=DIRECTION('ref_axis',(1.35391388547336E-32,1.,-1.21271509589043E-15));
#8494=DIRECTION('center_axis',(-6.46977897737062E-17,1.35628725133693E-15,
-1.));
#8495=DIRECTION('ref_axis',(2.45620303514854E-34,1.,1.35628725133693E-15));
#8496=DIRECTION('center_axis',(0.,0.,1.));
#8497=DIRECTION('ref_axis',(1.,0.,0.));
#8498=DIRECTION('center_axis',(0.,0.,-1.));
#8499=DIRECTION('ref_axis',(-1.,0.,0.));
#8500=DIRECTION('center_axis',(0.,0.,1.));
#8501=DIRECTION('ref_axis',(1.,0.,0.));
#8502=DIRECTION('center_axis',(0.,0.,-1.));
#8503=DIRECTION('ref_axis',(-1.,0.,0.));
#8504=DIRECTION('center_axis',(2.18703987820102E-16,1.34010054766509E-15,
-1.));
#8505=DIRECTION('ref_axis',(2.70980336596319E-33,1.,1.34010054766509E-15));
#8506=DIRECTION('center_axis',(0.,0.,1.));
#8507=DIRECTION('ref_axis',(1.,0.,0.));
#8508=DIRECTION('center_axis',(0.,0.,-1.));
#8509=DIRECTION('ref_axis',(-1.,0.,0.));
#8510=DIRECTION('center_axis',(0.,0.,1.));
#8511=DIRECTION('ref_axis',(1.,0.,0.));
#8512=DIRECTION('center_axis',(0.,0.,-1.));
#8513=DIRECTION('ref_axis',(-1.,0.,0.));
#8514=DIRECTION('center_axis',(4.92547351688005E-16,1.2653450195444E-15,
-1.));
#8515=DIRECTION('ref_axis',(1.39597070338658E-32,1.,1.2653450195444E-15));
#8516=DIRECTION('center_axis',(2.50582917348385E-16,-2.16552109648485E-15,
1.));
#8517=DIRECTION('ref_axis',(6.10963913452889E-32,-1.,-2.16552109648485E-15));
#8518=DIRECTION('center_axis',(0.,0.,-1.));
#8519=DIRECTION('ref_axis',(-1.,0.,0.));
#8520=DIRECTION('center_axis',(0.,0.,1.));
#8521=DIRECTION('ref_axis',(1.,0.,0.));
#8522=DIRECTION('center_axis',(-1.2069281093736E-15,-6.22113696155711E-16,
-1.));
#8523=DIRECTION('ref_axis',(-1.,-1.73910758130846E-32,1.2069281093736E-15));
#8524=DIRECTION('center_axis',(0.,0.,-1.));
#8525=DIRECTION('ref_axis',(-1.,0.,0.));
#8526=DIRECTION('center_axis',(0.,0.,1.));
#8527=DIRECTION('ref_axis',(1.,0.,0.));
#8528=DIRECTION('center_axis',(0.,0.,-1.));
#8529=DIRECTION('ref_axis',(-1.,0.,0.));
#8530=DIRECTION('center_axis',(0.,0.,1.));
#8531=DIRECTION('ref_axis',(1.,0.,0.));
#8532=DIRECTION('center_axis',(0.,0.,-1.));
#8533=DIRECTION('ref_axis',(-1.,0.,0.));
#8534=DIRECTION('center_axis',(9.64626581390641E-16,9.5561313857402E-16,
-1.));
#8535=DIRECTION('ref_axis',(-1.,2.270861517335E-32,-9.64626581390641E-16));
#8536=DIRECTION('center_axis',(0.,0.,1.));
#8537=DIRECTION('ref_axis',(1.,0.,0.));
#8538=DIRECTION('center_axis',(0.,0.,-1.));
#8539=DIRECTION('ref_axis',(-1.,0.,0.));
#8540=DIRECTION('center_axis',(0.,0.,1.));
#8541=DIRECTION('ref_axis',(1.,0.,0.));
#8542=DIRECTION('center_axis',(-1.35562012840529E-15,-7.74272536198608E-17,
-1.));
#8543=DIRECTION('ref_axis',(-1.,2.42293261278864E-34,1.35562012840529E-15));
#8544=DIRECTION('center_axis',(1.1422303195999E-15,7.34173555181198E-16,
-1.));
#8545=DIRECTION('ref_axis',(-1.,1.83215133257466E-32,-1.1422303195999E-15));
#8546=DIRECTION('center_axis',(0.,0.,1.));
#8547=DIRECTION('ref_axis',(1.,0.,0.));
#8548=DIRECTION('center_axis',(0.,0.,-1.));
#8549=DIRECTION('ref_axis',(-1.,0.,0.));
#8550=DIRECTION('center_axis',(0.,0.,1.));
#8551=DIRECTION('ref_axis',(1.,0.,0.));
#8552=DIRECTION('center_axis',(0.,0.,-1.));
#8553=DIRECTION('ref_axis',(-1.,0.,0.));
#8554=DIRECTION('center_axis',(0.,0.,-1.));
#8555=DIRECTION('ref_axis',(-1.,0.,0.));
#8556=DIRECTION('center_axis',(0.,0.,1.));
#8557=DIRECTION('ref_axis',(1.,0.,0.));
#8558=DIRECTION('center_axis',(0.,0.,-1.));
#8559=DIRECTION('ref_axis',(-1.,0.,0.));
#8560=DIRECTION('center_axis',(0.,0.,1.));
#8561=DIRECTION('ref_axis',(1.,0.,0.));
#8562=DIRECTION('center_axis',(0.,0.,-1.));
#8563=DIRECTION('ref_axis',(-1.,0.,0.));
#8564=DIRECTION('center_axis',(0.,0.,-1.));
#8565=DIRECTION('ref_axis',(-1.,0.,0.));
#8566=DIRECTION('center_axis',(1.0701355254071E-15,-1.89923231202752E-15,
1.));
#8567=DIRECTION('ref_axis',(-3.13557062175357E-31,-1.,-1.89923231202752E-15));
#8568=DIRECTION('center_axis',(0.,0.,-1.));
#8569=DIRECTION('ref_axis',(-1.,0.,0.));
#8570=DIRECTION('center_axis',(0.,0.,-1.));
#8571=DIRECTION('ref_axis',(-1.,0.,0.));
#8572=DIRECTION('center_axis',(0.,0.,1.));
#8573=DIRECTION('ref_axis',(1.,0.,0.));
#8574=DIRECTION('center_axis',(-9.64626581390635E-16,9.55613138574038E-16,
-1.));
#8575=DIRECTION('ref_axis',(-1.,-2.27086151733484E-32,9.64626581390635E-16));
#8576=DIRECTION('center_axis',(0.,0.,-1.));
#8577=DIRECTION('ref_axis',(-1.,0.,0.));
#8578=DIRECTION('center_axis',(0.,0.,-1.));
#8579=DIRECTION('ref_axis',(-1.,0.,0.));
#8580=DIRECTION('center_axis',(0.,0.,1.));
#8581=DIRECTION('ref_axis',(1.,0.,0.));
#8582=DIRECTION('center_axis',(-7.44864032782697E-16,1.13528784227057E-15,
-1.));
#8583=DIRECTION('ref_axis',(1.34170956239683E-32,1.,1.13528784227057E-15));
#8584=DIRECTION('center_axis',(0.,0.,-1.));
#8585=DIRECTION('ref_axis',(-1.,0.,0.));
#8586=DIRECTION('center_axis',(0.,0.,-1.));
#8587=DIRECTION('ref_axis',(-1.,0.,0.));
#8588=DIRECTION('center_axis',(-2.50582917348388E-16,-2.16552109648484E-15,
1.));
#8589=DIRECTION('ref_axis',(-6.10963913452999E-32,-1.,-2.16552109648484E-15));
#8590=DIRECTION('center_axis',(0.,0.,-1.));
#8591=DIRECTION('ref_axis',(-1.,0.,0.));
#8592=DIRECTION('center_axis',(1.05120912399335E-15,-8.59453483193718E-16,
-1.));
#8593=DIRECTION('ref_axis',(-1.,6.24131468909447E-33,-1.05120912399335E-15));
#8594=DIRECTION('center_axis',(0.,0.,-1.));
#8595=DIRECTION('ref_axis',(-1.,0.,0.));
#8596=DIRECTION('center_axis',(0.,0.,1.));
#8597=DIRECTION('ref_axis',(1.,0.,0.));
#8598=DIRECTION('center_axis',(-2.18703987820084E-16,1.34010054766509E-15,
-1.));
#8599=DIRECTION('ref_axis',(-2.70980336596201E-33,1.,1.34010054766509E-15));
#8600=DIRECTION('center_axis',(0.,0.,-1.));
#8601=DIRECTION('ref_axis',(-1.,0.,0.));
#8602=DIRECTION('center_axis',(0.,0.,-1.));
#8603=DIRECTION('ref_axis',(-1.,0.,0.));
#8604=DIRECTION('center_axis',(0.,0.,1.));
#8605=DIRECTION('ref_axis',(1.,0.,0.));
#8606=DIRECTION('center_axis',(0.,0.,-1.));
#8607=DIRECTION('ref_axis',(-1.,0.,0.));
#8608=DIRECTION('center_axis',(6.10756095622563E-16,-1.21271509589044E-15,
-1.));
#8609=DIRECTION('ref_axis',(-1.35391388547399E-32,1.,-1.21271509589044E-15));
#8610=DIRECTION('center_axis',(0.,0.,-1.));
#8611=DIRECTION('ref_axis',(-1.,0.,0.));
#8612=DIRECTION('center_axis',(0.,0.,1.));
#8613=DIRECTION('ref_axis',(1.,0.,0.));
#8614=DIRECTION('center_axis',(3.45271963499982E-16,1.31319769393704E-15,
-1.));
#8615=DIRECTION('ref_axis',(-6.73653793160646E-33,1.,1.31319769393704E-15));
#8616=DIRECTION('center_axis',(0.,0.,-1.));
#8617=DIRECTION('ref_axis',(-1.,0.,0.));
#8618=DIRECTION('center_axis',(0.,0.,1.));
#8619=DIRECTION('ref_axis',(1.,0.,0.));
#8620=DIRECTION('center_axis',(0.,0.,-1.));
#8621=DIRECTION('ref_axis',(-1.,0.,0.));
#8622=DIRECTION('center_axis',(0.,0.,-1.));
#8623=DIRECTION('ref_axis',(-1.,0.,0.));
#8624=DIRECTION('center_axis',(6.4697789773697E-17,-1.35628725133693E-15,
-1.));
#8625=DIRECTION('ref_axis',(2.45620303515335E-34,1.,-1.35628725133693E-15));
#8626=DIRECTION('center_axis',(0.,0.,1.));
#8627=DIRECTION('ref_axis',(1.,0.,0.));
#8628=DIRECTION('center_axis',(0.,0.,-1.));
#8629=DIRECTION('ref_axis',(-1.,0.,0.));
#8630=DIRECTION('center_axis',(8.49547255633585E-16,1.05923102890075E-15,
-1.));
#8631=DIRECTION('ref_axis',(-6.4561121370934E-34,1.,1.05923102890075E-15));
#8632=DIRECTION('center_axis',(0.,0.,-1.));
#8633=DIRECTION('ref_axis',(-1.,0.,0.));
#8634=DIRECTION('center_axis',(0.,0.,1.));
#8635=DIRECTION('ref_axis',(1.,0.,0.));
#8636=DIRECTION('center_axis',(0.,0.,-1.));
#8637=DIRECTION('ref_axis',(-1.,0.,0.));
#8638=DIRECTION('center_axis',(0.,0.,-1.));
#8639=DIRECTION('ref_axis',(-1.,0.,0.));
#8640=DIRECTION('center_axis',(-4.92547351688011E-16,-1.26534501954439E-15,
-1.));
#8641=DIRECTION('ref_axis',(1.39597070338681E-32,1.,-1.26534501954439E-15));
#8642=DIRECTION('center_axis',(0.,0.,1.));
#8643=DIRECTION('ref_axis',(1.,0.,0.));
#8644=DIRECTION('center_axis',(0.,0.,-1.));
#8645=DIRECTION('ref_axis',(-1.,0.,0.));
#8646=DIRECTION('center_axis',(0.,0.,-1.));
#8647=DIRECTION('ref_axis',(-1.,0.,0.));
#8648=DIRECTION('center_axis',(-7.44864032782725E-16,-1.13528784227056E-15,
-1.));
#8649=DIRECTION('ref_axis',(-1.3417095623968E-32,1.,-1.13528784227056E-15));
#8650=DIRECTION('center_axis',(0.,0.,1.));
#8651=DIRECTION('ref_axis',(1.,0.,0.));
#8652=DIRECTION('center_axis',(0.,0.,-1.));
#8653=DIRECTION('ref_axis',(-1.,0.,0.));
#8654=DIRECTION('center_axis',(0.,0.,-1.));
#8655=DIRECTION('ref_axis',(-1.,0.,0.));
#8656=DIRECTION('center_axis',(0.,0.,-1.));
#8657=DIRECTION('ref_axis',(-1.,0.,0.));
#8658=DIRECTION('center_axis',(0.,0.,1.));
#8659=DIRECTION('ref_axis',(1.,0.,0.));
#8660=DIRECTION('center_axis',(0.,0.,-1.));
#8661=DIRECTION('ref_axis',(-1.,0.,0.));
#8662=DIRECTION('center_axis',(-1.14223031959991E-15,-7.34173555181192E-16,
-1.));
#8663=DIRECTION('ref_axis',(-1.,1.83215133257436E-32,1.14223031959991E-15));
#8664=DIRECTION('center_axis',(0.,0.,1.));
#8665=DIRECTION('ref_axis',(1.,0.,0.));
#8666=DIRECTION('center_axis',(0.,0.,-1.));
#8667=DIRECTION('ref_axis',(-1.,0.,0.));
#8668=DIRECTION('center_axis',(-4.15432588173314E-15,3.95257705004225E-14,
1.));
#8669=DIRECTION('ref_axis',(1.01104027505707E-32,-1.,3.95257705004225E-14));
#8670=DIRECTION('center_axis',(-1.26991311181345E-15,-4.80647064471381E-16,
-1.));
#8671=DIRECTION('ref_axis',(-1.,-1.14267906456524E-32,1.26991311181345E-15));
#8672=DIRECTION('center_axis',(0.,0.,1.));
#8673=DIRECTION('ref_axis',(1.,0.,0.));
#8674=DIRECTION('center_axis',(0.,0.,-1.));
#8675=DIRECTION('ref_axis',(-1.,0.,0.));
#8676=DIRECTION('center_axis',(0.,0.,1.));
#8677=DIRECTION('ref_axis',(1.,0.,0.));
#8678=DIRECTION('center_axis',(0.,0.,-1.));
#8679=DIRECTION('ref_axis',(-1.,0.,0.));
#8680=DIRECTION('center_axis',(0.,0.,-1.));
#8681=DIRECTION('ref_axis',(-1.,0.,0.));
#8682=DIRECTION('center_axis',(0.,0.,1.));
#8683=DIRECTION('ref_axis',(1.,0.,0.));
#8684=DIRECTION('center_axis',(0.,0.,-1.));
#8685=DIRECTION('ref_axis',(-1.,0.,0.));
#8686=DIRECTION('center_axis',(0.,0.,1.));
#8687=DIRECTION('ref_axis',(1.,0.,0.));
#8688=DIRECTION('center_axis',(0.,0.,-1.));
#8689=DIRECTION('ref_axis',(-1.,0.,0.));
#8690=DIRECTION('center_axis',(-1.35562012840529E-15,7.74272536198692E-17,
-1.));
#8691=DIRECTION('ref_axis',(-1.,-2.42293261278252E-34,1.35562012840529E-15));
#8692=DIRECTION('center_axis',(0.,0.,1.));
#8693=DIRECTION('ref_axis',(1.,0.,0.));
#8694=DIRECTION('center_axis',(0.,0.,-1.));
#8695=DIRECTION('ref_axis',(-1.,0.,0.));
#8696=DIRECTION('center_axis',(0.,0.,1.));
#8697=DIRECTION('ref_axis',(1.,0.,0.));
#8698=DIRECTION('center_axis',(0.,0.,-1.));
#8699=DIRECTION('ref_axis',(-1.,0.,0.));
#8700=DIRECTION('center_axis',(-1.3098985448906E-15,3.57584555363018E-16,
-1.));
#8701=DIRECTION('ref_axis',(-1.,-5.79704190756504E-33,1.3098985448906E-15));
#8702=DIRECTION('center_axis',(0.,0.,1.));
#8703=DIRECTION('ref_axis',(1.,0.,0.));
#8704=DIRECTION('center_axis',(0.,0.,-1.));
#8705=DIRECTION('ref_axis',(-1.,0.,0.));
#8706=DIRECTION('center_axis',(0.,0.,1.));
#8707=DIRECTION('ref_axis',(1.,0.,0.));
#8708=DIRECTION('center_axis',(0.,0.,-1.));
#8709=DIRECTION('ref_axis',(-1.,0.,0.));
#8710=DIRECTION('',(0.,-1.,0.));
#8711=DIRECTION('',(0.,1.,0.));
#8712=DIRECTION('',(-1.,0.,0.));
#8713=DIRECTION('center_axis',(0.,0.,1.));
#8714=DIRECTION('ref_axis',(1.,0.,0.));
#8715=DIRECTION('center_axis',(0.,0.,-1.));
#8716=DIRECTION('ref_axis',(-1.,0.,0.));
#8717=DIRECTION('center_axis',(-7.4486403278271E-16,1.13528784227057E-15,
-1.));
#8718=DIRECTION('ref_axis',(1.34170956239694E-32,1.,1.13528784227057E-15));
#8719=DIRECTION('center_axis',(0.,0.,-1.));
#8720=DIRECTION('ref_axis',(-1.,0.,0.));
#8721=DIRECTION('center_axis',(0.,0.,-1.));
#8722=DIRECTION('ref_axis',(-1.,0.,0.));
#8723=DIRECTION('center_axis',(0.,0.,-1.));
#8724=DIRECTION('ref_axis',(-1.,0.,0.));
#8725=DIRECTION('center_axis',(0.,0.,-1.));
#8726=DIRECTION('ref_axis',(-1.,0.,0.));
#8727=DIRECTION('center_axis',(0.,0.,-1.));
#8728=DIRECTION('ref_axis',(-1.,0.,0.));
#8729=DIRECTION('center_axis',(0.,0.,-1.));
#8730=DIRECTION('ref_axis',(-1.,0.,0.));
#8731=DIRECTION('center_axis',(0.,0.,-1.));
#8732=DIRECTION('ref_axis',(-1.,0.,0.));
#8733=DIRECTION('center_axis',(0.,0.,-1.));
#8734=DIRECTION('ref_axis',(-1.,0.,0.));
#8735=DIRECTION('center_axis',(1.35562012840529E-15,-7.74272536198712E-17,
-1.));
#8736=DIRECTION('ref_axis',(-1.,-2.42293261278146E-34,-1.35562012840529E-15));
#8737=DIRECTION('center_axis',(-1.1422303195999E-15,7.34173555181211E-16,
-1.));
#8738=DIRECTION('ref_axis',(-1.,-1.83215133257424E-32,1.1422303195999E-15));
#8739=DIRECTION('center_axis',(0.,0.,-1.));
#8740=DIRECTION('ref_axis',(-1.,0.,0.));
#8741=DIRECTION('center_axis',(0.,0.,-1.));
#8742=DIRECTION('ref_axis',(-1.,0.,0.));
#8743=DIRECTION('center_axis',(0.,0.,-1.));
#8744=DIRECTION('ref_axis',(-1.,0.,0.));
#8745=DIRECTION('center_axis',(1.34209460732158E-15,2.0611399064365E-16,
-1.));
#8746=DIRECTION('ref_axis',(-1.,-2.1428061985013E-33,-1.34209460732158E-15));
#8747=DIRECTION('center_axis',(0.,0.,-1.));
#8748=DIRECTION('ref_axis',(-1.,0.,0.));
#8749=DIRECTION('center_axis',(0.,0.,-1.));
#8750=DIRECTION('ref_axis',(-1.,0.,0.));
#8751=DIRECTION('center_axis',(0.,0.,-1.));
#8752=DIRECTION('ref_axis',(-1.,0.,0.));
#8753=DIRECTION('center_axis',(0.,0.,-1.));
#8754=DIRECTION('ref_axis',(-1.,0.,0.));
#8755=DIRECTION('center_axis',(0.,0.,-1.));
#8756=DIRECTION('ref_axis',(-1.,0.,0.));
#8757=DIRECTION('center_axis',(4.15432588173204E-15,-3.95257705004099E-14,
1.));
#8758=DIRECTION('ref_axis',(1.011040284911E-32,-1.,-3.95257705004099E-14));
#8759=DIRECTION('center_axis',(0.,0.,-1.));
#8760=DIRECTION('ref_axis',(-1.,0.,0.));
#8761=DIRECTION('center_axis',(0.,0.,-1.));
#8762=DIRECTION('ref_axis',(-1.,0.,0.));
#8763=DIRECTION('center_axis',(0.,0.,-1.));
#8764=DIRECTION('ref_axis',(-1.,0.,0.));
#8765=DIRECTION('center_axis',(0.,0.,-1.));
#8766=DIRECTION('ref_axis',(-1.,0.,0.));
#8767=DIRECTION('center_axis',(0.,0.,-1.));
#8768=DIRECTION('ref_axis',(-1.,0.,0.));
#8769=DIRECTION('center_axis',(0.,0.,-1.));
#8770=DIRECTION('ref_axis',(-1.,0.,0.));
#8771=DIRECTION('center_axis',(0.,0.,-1.));
#8772=DIRECTION('ref_axis',(-1.,0.,0.));
#8773=DIRECTION('center_axis',(0.,0.,-1.));
#8774=DIRECTION('ref_axis',(-1.,0.,0.));
#8775=DIRECTION('center_axis',(0.,0.,-1.));
#8776=DIRECTION('ref_axis',(-1.,0.,0.));
#8777=DIRECTION('center_axis',(7.44864032782723E-16,1.13528784227056E-15,
-1.));
#8778=DIRECTION('ref_axis',(-1.34170956239609E-32,1.,1.13528784227056E-15));
#8779=DIRECTION('center_axis',(0.,0.,-1.));
#8780=DIRECTION('ref_axis',(-1.,0.,0.));
#8781=DIRECTION('center_axis',(0.,0.,-1.));
#8782=DIRECTION('ref_axis',(-1.,0.,0.));
#8783=DIRECTION('center_axis',(0.,0.,-1.));
#8784=DIRECTION('ref_axis',(-1.,0.,0.));
#8785=DIRECTION('center_axis',(0.,0.,-1.));
#8786=DIRECTION('ref_axis',(-1.,0.,0.));
#8787=DIRECTION('center_axis',(0.,0.,-1.));
#8788=DIRECTION('ref_axis',(-1.,0.,0.));
#8789=DIRECTION('center_axis',(0.,0.,-1.));
#8790=DIRECTION('ref_axis',(-1.,0.,0.));
#8791=DIRECTION('center_axis',(0.,0.,-1.));
#8792=DIRECTION('ref_axis',(-1.,0.,0.));
#8793=DIRECTION('center_axis',(0.,0.,-1.));
#8794=DIRECTION('ref_axis',(-1.,0.,0.));
#8795=DIRECTION('center_axis',(0.,0.,-1.));
#8796=DIRECTION('ref_axis',(-1.,0.,0.));
#8797=DIRECTION('center_axis',(0.,0.,-1.));
#8798=DIRECTION('ref_axis',(-1.,0.,0.));
#8799=DIRECTION('center_axis',(0.,0.,-1.));
#8800=DIRECTION('ref_axis',(-1.,0.,0.));
#8801=DIRECTION('center_axis',(-6.46977897736951E-17,1.35628725133693E-15,
-1.));
#8802=DIRECTION('ref_axis',(2.4562030351539E-34,1.,1.35628725133693E-15));
#8803=DIRECTION('center_axis',(-6.10756095622592E-16,-1.21271509589044E-15,
-1.));
#8804=DIRECTION('ref_axis',(1.35391388547316E-32,1.,-1.21271509589044E-15));
#8805=DIRECTION('center_axis',(0.,0.,-1.));
#8806=DIRECTION('ref_axis',(-1.,0.,0.));
#8807=DIRECTION('center_axis',(0.,0.,-1.));
#8808=DIRECTION('ref_axis',(-1.,0.,0.));
#8809=DIRECTION('center_axis',(0.,0.,-1.));
#8810=DIRECTION('ref_axis',(-1.,0.,0.));
#8811=DIRECTION('center_axis',(-3.45271963499982E-16,-1.31319769393704E-15,
-1.));
#8812=DIRECTION('ref_axis',(-6.73653793160646E-33,1.,-1.31319769393704E-15));
#8813=DIRECTION('center_axis',(0.,0.,-1.));
#8814=DIRECTION('ref_axis',(-1.,0.,0.));
#8815=DIRECTION('center_axis',(0.,0.,-1.));
#8816=DIRECTION('ref_axis',(-1.,0.,0.));
#8817=DIRECTION('center_axis',(0.,0.,-1.));
#8818=DIRECTION('ref_axis',(-1.,0.,0.));
#8819=DIRECTION('center_axis',(-6.46977897737243E-17,-1.35628725133692E-15,
-1.));
#8820=DIRECTION('ref_axis',(-2.45620303514865E-34,1.,-1.35628725133692E-15));
#8821=DIRECTION('center_axis',(0.,0.,-1.));
#8822=DIRECTION('ref_axis',(-1.,0.,0.));
#8823=DIRECTION('center_axis',(0.,0.,-1.));
#8824=DIRECTION('ref_axis',(-1.,0.,0.));
#8825=DIRECTION('center_axis',(0.,0.,-1.));
#8826=DIRECTION('ref_axis',(-1.,0.,0.));
#8827=DIRECTION('center_axis',(2.18703987820084E-16,-1.34010054766509E-15,
-1.));
#8828=DIRECTION('ref_axis',(-2.70980336596175E-33,1.,-1.34010054766509E-15));
#8829=DIRECTION('center_axis',(0.,0.,-1.));
#8830=DIRECTION('ref_axis',(-1.,0.,0.));
#8831=DIRECTION('center_axis',(0.,0.,-1.));
#8832=DIRECTION('ref_axis',(-1.,0.,0.));
#8833=DIRECTION('center_axis',(0.,0.,-1.));
#8834=DIRECTION('ref_axis',(-1.,0.,0.));
#8835=DIRECTION('center_axis',(4.92547351687991E-16,-1.26534501954442E-15,
-1.));
#8836=DIRECTION('ref_axis',(-1.39597070338527E-32,1.,-1.26534501954442E-15));
#8837=DIRECTION('center_axis',(-2.50582917348388E-16,-2.16552109648484E-15,
-1.));
#8838=DIRECTION('ref_axis',(6.10963913452999E-32,1.,-2.16552109648484E-15));
#8839=DIRECTION('center_axis',(0.,0.,-1.));
#8840=DIRECTION('ref_axis',(-1.,0.,0.));
#8841=DIRECTION('center_axis',(-1.2069281093736E-15,6.22113696155734E-16,
-1.));
#8842=DIRECTION('ref_axis',(-1.,1.73910758130861E-32,1.2069281093736E-15));
#8843=DIRECTION('center_axis',(7.44864032782693E-16,-1.13528784227057E-15,
-1.));
#8844=DIRECTION('ref_axis',(1.34170956239657E-32,1.,-1.13528784227057E-15));
#8845=DIRECTION('center_axis',(0.,0.,-1.));
#8846=DIRECTION('ref_axis',(-1.,0.,0.));
#8847=DIRECTION('center_axis',(0.,0.,-1.));
#8848=DIRECTION('ref_axis',(-1.,0.,0.));
#8849=DIRECTION('center_axis',(0.,0.,-1.));
#8850=DIRECTION('ref_axis',(-1.,0.,0.));
#8851=DIRECTION('center_axis',(0.,0.,-1.));
#8852=DIRECTION('ref_axis',(-1.,0.,0.));
#8853=DIRECTION('center_axis',(0.,0.,-1.));
#8854=DIRECTION('ref_axis',(-1.,0.,0.));
#8855=DIRECTION('center_axis',(0.,0.,-1.));
#8856=DIRECTION('ref_axis',(-1.,0.,0.));
#8857=DIRECTION('center_axis',(0.,0.,-1.));
#8858=DIRECTION('ref_axis',(-1.,0.,0.));
#8859=DIRECTION('center_axis',(1.0701355254071E-15,-1.89923231202752E-15,
-1.));
#8860=DIRECTION('ref_axis',(3.13557062175357E-31,1.,-1.89923231202752E-15));
#8861=DIRECTION('center_axis',(0.,0.,-1.));
#8862=DIRECTION('ref_axis',(-1.,0.,0.));
#8863=DIRECTION('center_axis',(1.26991311181345E-15,-4.80647064471377E-16,
-1.));
#8864=DIRECTION('ref_axis',(-1.,1.14267906456546E-32,-1.26991311181345E-15));
#8865=DIRECTION('center_axis',(0.,0.,-1.));
#8866=DIRECTION('ref_axis',(-1.,0.,0.));
#8867=DIRECTION('center_axis',(0.,0.,-1.));
#8868=DIRECTION('ref_axis',(-1.,0.,0.));
#8869=DIRECTION('center_axis',(0.,0.,-1.));
#8870=DIRECTION('ref_axis',(-1.,0.,0.));
#8871=DIRECTION('center_axis',(0.,0.,-1.));
#8872=DIRECTION('ref_axis',(-1.,0.,0.));
#8873=DIRECTION('center_axis',(0.,0.,-1.));
#8874=DIRECTION('ref_axis',(-1.,0.,0.));
#8875=DIRECTION('center_axis',(0.,0.,-1.));
#8876=DIRECTION('ref_axis',(-1.,0.,0.));
#8877=DIRECTION('center_axis',(0.,0.,-1.));
#8878=DIRECTION('ref_axis',(-1.,0.,0.));
#8879=DIRECTION('center_axis',(0.,0.,-1.));
#8880=DIRECTION('ref_axis',(-1.,0.,0.));
#8881=DIRECTION('center_axis',(0.,0.,-1.));
#8882=DIRECTION('ref_axis',(-1.,0.,0.));
#8883=DIRECTION('center_axis',(1.35562012840529E-15,7.74272536198596E-17,
-1.));
#8884=DIRECTION('ref_axis',(-1.,2.42293261278592E-34,-1.35562012840529E-15));
#8885=DIRECTION('center_axis',(0.,0.,-1.));
#8886=DIRECTION('ref_axis',(-1.,0.,0.));
#8887=DIRECTION('center_axis',(0.,0.,-1.));
#8888=DIRECTION('ref_axis',(-1.,0.,0.));
#8889=DIRECTION('center_axis',(0.,0.,-1.));
#8890=DIRECTION('ref_axis',(-1.,0.,0.));
#8891=DIRECTION('center_axis',(0.,0.,-1.));
#8892=DIRECTION('ref_axis',(-1.,0.,0.));
#8893=DIRECTION('center_axis',(1.3098985448906E-15,3.57584555363002E-16,
-1.));
#8894=DIRECTION('ref_axis',(-1.,5.79704190755911E-33,-1.3098985448906E-15));
#8895=DIRECTION('center_axis',(0.,0.,-1.));
#8896=DIRECTION('ref_axis',(-1.,0.,0.));
#8897=DIRECTION('center_axis',(0.,0.,-1.));
#8898=DIRECTION('ref_axis',(-1.,0.,0.));
#8899=DIRECTION('center_axis',(0.,0.,-1.));
#8900=DIRECTION('ref_axis',(-1.,0.,0.));
#8901=DIRECTION('center_axis',(0.,0.,-1.));
#8902=DIRECTION('ref_axis',(-1.,0.,0.));
#8903=DIRECTION('center_axis',(1.2069281093736E-15,6.22113696155711E-16,
-1.));
#8904=DIRECTION('ref_axis',(-1.,-1.73910758130838E-32,-1.2069281093736E-15));
#8905=DIRECTION('center_axis',(0.,0.,-1.));
#8906=DIRECTION('ref_axis',(-1.,0.,0.));
#8907=DIRECTION('center_axis',(0.,0.,-1.));
#8908=DIRECTION('ref_axis',(-1.,0.,0.));
#8909=DIRECTION('center_axis',(2.50582917348385E-16,-2.16552109648485E-15,
-1.));
#8910=DIRECTION('ref_axis',(-6.10963913452889E-32,1.,-2.16552109648485E-15));
#8911=DIRECTION('center_axis',(0.,0.,-1.));
#8912=DIRECTION('ref_axis',(-1.,0.,0.));
#8913=DIRECTION('center_axis',(0.,0.,-1.));
#8914=DIRECTION('ref_axis',(-1.,0.,0.));
#8915=DIRECTION('center_axis',(0.,0.,-1.));
#8916=DIRECTION('ref_axis',(-1.,0.,0.));
#8917=DIRECTION('center_axis',(0.,0.,-1.));
#8918=DIRECTION('ref_axis',(-1.,0.,0.));
#8919=DIRECTION('center_axis',(0.,0.,-1.));
#8920=DIRECTION('ref_axis',(-1.,0.,0.));
#8921=DIRECTION('center_axis',(0.,0.,-1.));
#8922=DIRECTION('ref_axis',(-1.,0.,0.));
#8923=DIRECTION('center_axis',(0.,0.,-1.));
#8924=DIRECTION('ref_axis',(-1.,0.,0.));
#8925=DIRECTION('center_axis',(0.,0.,-1.));
#8926=DIRECTION('ref_axis',(-1.,0.,0.));
#8927=DIRECTION('center_axis',(0.,0.,-1.));
#8928=DIRECTION('ref_axis',(-1.,0.,0.));
#8929=DIRECTION('center_axis',(0.,0.,-1.));
#8930=DIRECTION('ref_axis',(-1.,0.,0.));
#8931=DIRECTION('center_axis',(0.,0.,-1.));
#8932=DIRECTION('ref_axis',(-1.,0.,0.));
#8933=DIRECTION('center_axis',(6.10756095622582E-16,1.21271509589044E-15,
-1.));
#8934=DIRECTION('ref_axis',(1.35391388547304E-32,1.,1.21271509589044E-15));
#8935=DIRECTION('center_axis',(0.,0.,-1.));
#8936=DIRECTION('ref_axis',(-1.,0.,0.));
#8937=DIRECTION('center_axis',(0.,0.,-1.));
#8938=DIRECTION('ref_axis',(-1.,0.,0.));
#8939=DIRECTION('center_axis',(0.,0.,-1.));
#8940=DIRECTION('ref_axis',(-1.,0.,0.));
#8941=DIRECTION('center_axis',(0.,0.,-1.));
#8942=DIRECTION('ref_axis',(-1.,0.,0.));
#8943=DIRECTION('center_axis',(0.,0.,-1.));
#8944=DIRECTION('ref_axis',(-1.,0.,0.));
#8945=DIRECTION('center_axis',(1.47558720267693E-15,1.6046544254399E-15,
-1.));
#8946=DIRECTION('ref_axis',(2.31817004142331E-33,1.,1.6046544254399E-15));
#8947=DIRECTION('center_axis',(0.,0.,-1.));
#8948=DIRECTION('ref_axis',(-1.,0.,0.));
#8949=DIRECTION('center_axis',(1.77696849674338E-15,-1.26279704599333E-15,
-1.));
#8950=DIRECTION('ref_axis',(-1.,-2.1561382677115E-31,-1.77696849674338E-15));
#8951=DIRECTION('center_axis',(0.,0.,-1.));
#8952=DIRECTION('ref_axis',(-1.,0.,0.));
#8953=DIRECTION('center_axis',(6.46977897737148E-17,1.35628725133693E-15,
-1.));
#8954=DIRECTION('ref_axis',(-2.45620303515642E-34,1.,1.35628725133693E-15));
#8955=DIRECTION('center_axis',(0.,0.,-1.));
#8956=DIRECTION('ref_axis',(-1.,0.,0.));
#8957=DIRECTION('center_axis',(0.,0.,-1.));
#8958=DIRECTION('ref_axis',(-1.,0.,0.));
#8959=DIRECTION('center_axis',(0.,0.,-1.));
#8960=DIRECTION('ref_axis',(-1.,0.,0.));
#8961=DIRECTION('center_axis',(0.,0.,-1.));
#8962=DIRECTION('ref_axis',(-1.,0.,0.));
#8963=DIRECTION('center_axis',(-2.18703987820093E-16,1.34010054766509E-15,
-1.));
#8964=DIRECTION('ref_axis',(-2.70980336596394E-33,1.,1.34010054766509E-15));
#8965=DIRECTION('center_axis',(0.,0.,-1.));
#8966=DIRECTION('ref_axis',(-1.,0.,0.));
#8967=DIRECTION('center_axis',(0.,0.,-1.));
#8968=DIRECTION('ref_axis',(-1.,0.,0.));
#8969=DIRECTION('center_axis',(0.,0.,-1.));
#8970=DIRECTION('ref_axis',(-1.,0.,0.));
#8971=DIRECTION('center_axis',(0.,0.,-1.));
#8972=DIRECTION('ref_axis',(-1.,0.,0.));
#8973=DIRECTION('center_axis',(0.,0.,-1.));
#8974=DIRECTION('ref_axis',(-1.,0.,0.));
#8975=DIRECTION('center_axis',(0.,0.,-1.));
#8976=DIRECTION('ref_axis',(-1.,0.,0.));
#8977=DIRECTION('center_axis',(0.,0.,-1.));
#8978=DIRECTION('ref_axis',(-1.,0.,0.));
#8979=DIRECTION('center_axis',(2.17985119260763E-15,2.28516055189852E-17,
-1.));
#8980=DIRECTION('ref_axis',(-1.,-5.24414567525364E-33,-2.17985119260763E-15));
#8981=DIRECTION('',(0.,-1.,0.));
#8982=DIRECTION('',(-1.,0.,0.));
#8983=DIRECTION('',(0.,1.,0.));
#8984=DIRECTION('center_axis',(0.,0.,-1.));
#8985=DIRECTION('ref_axis',(-1.,0.,0.));
#8986=DIRECTION('',(0.,0.,-1.));
#8987=DIRECTION('center_axis',(0.,0.,1.));
#8988=DIRECTION('ref_axis',(1.,0.,0.));
#8989=DIRECTION('',(0.,0.,1.));
#8990=DIRECTION('center_axis',(0.,0.,1.));
#8991=DIRECTION('ref_axis',(1.,0.,0.));
#8992=DIRECTION('',(0.,0.,-1.));
#8993=DIRECTION('center_axis',(0.,0.,1.));
#8994=DIRECTION('ref_axis',(1.,0.,0.));
#8995=DIRECTION('',(0.,0.,-1.));
#8996=DIRECTION('',(0.,0.,1.));
#8997=DIRECTION('center_axis',(0.,0.,-1.));
#8998=DIRECTION('ref_axis',(-1.,0.,0.));
#8999=DIRECTION('center_axis',(0.,0.,-1.));
#9000=DIRECTION('ref_axis',(-1.,0.,0.));
#9001=DIRECTION('center_axis',(0.,0.,1.));
#9002=DIRECTION('ref_axis',(-0.988411742041742,-0.151796667269113,0.));
#9003=DIRECTION('',(0.,0.,-1.));
#9004=DIRECTION('center_axis',(0.,0.,1.));
#9005=DIRECTION('ref_axis',(1.,0.,0.));
#9006=DIRECTION('',(0.,0.,1.));
#9007=DIRECTION('center_axis',(0.,0.,-1.));
#9008=DIRECTION('ref_axis',(-1.,0.,0.));
#9009=DIRECTION('',(0.,0.,-1.));
#9010=DIRECTION('center_axis',(0.,0.,1.));
#9011=DIRECTION('ref_axis',(1.,0.,0.));
#9012=DIRECTION('',(0.,0.,1.));
#9013=DIRECTION('center_axis',(0.,0.,-1.));
#9014=DIRECTION('ref_axis',(0.802811069346196,0.596233500346314,0.));
#9015=DIRECTION('center_axis',(0.,0.,1.));
#9016=DIRECTION('ref_axis',(1.,0.,0.));
#9017=DIRECTION('center_axis',(0.,0.,1.));
#9018=DIRECTION('ref_axis',(1.,0.,0.));
#9019=DIRECTION('',(0.,0.,1.));
#9020=DIRECTION('center_axis',(0.,0.,-1.));
#9021=DIRECTION('ref_axis',(-1.,0.,0.));
#9022=DIRECTION('',(0.,0.,-1.));
#9023=DIRECTION('center_axis',(0.,0.,1.));
#9024=DIRECTION('ref_axis',(1.,0.,0.));
#9025=DIRECTION('center_axis',(0.,0.,1.));
#9026=DIRECTION('ref_axis',(1.,0.,0.));
#9027=DIRECTION('center_axis',(0.,0.,1.));
#9028=DIRECTION('ref_axis',(1.,0.,0.));
#9029=DIRECTION('',(0.,0.,1.));
#9030=DIRECTION('center_axis',(0.,0.,-1.));
#9031=DIRECTION('ref_axis',(-1.,0.,0.));
#9032=DIRECTION('',(0.,0.,-1.));
#9033=DIRECTION('center_axis',(0.,0.,1.));
#9034=DIRECTION('ref_axis',(1.,0.,0.));
#9035=DIRECTION('center_axis',(0.,0.,1.));
#9036=DIRECTION('ref_axis',(1.,0.,0.));
#9037=DIRECTION('center_axis',(0.,0.,1.));
#9038=DIRECTION('ref_axis',(1.,0.,0.));
#9039=DIRECTION('',(0.,0.,1.));
#9040=DIRECTION('center_axis',(0.,0.,-1.));
#9041=DIRECTION('ref_axis',(-1.,0.,0.));
#9042=DIRECTION('',(0.,0.,-1.));
#9043=DIRECTION('center_axis',(0.,0.,1.));
#9044=DIRECTION('ref_axis',(1.,0.,0.));
#9045=DIRECTION('center_axis',(0.,0.,1.));
#9046=DIRECTION('ref_axis',(1.,0.,0.));
#9047=DIRECTION('center_axis',(0.,0.,1.));
#9048=DIRECTION('ref_axis',(1.,0.,0.));
#9049=DIRECTION('',(0.,0.,1.));
#9050=DIRECTION('center_axis',(0.,0.,-1.));
#9051=DIRECTION('ref_axis',(-1.,0.,0.));
#9052=DIRECTION('',(0.,0.,-1.));
#9053=DIRECTION('center_axis',(0.,0.,1.));
#9054=DIRECTION('ref_axis',(1.,0.,0.));
#9055=DIRECTION('center_axis',(0.,0.,1.));
#9056=DIRECTION('ref_axis',(1.,0.,0.));
#9057=DIRECTION('center_axis',(0.,0.,1.));
#9058=DIRECTION('ref_axis',(1.,0.,0.));
#9059=DIRECTION('',(0.,0.,1.));
#9060=DIRECTION('center_axis',(0.,0.,-1.));
#9061=DIRECTION('ref_axis',(-1.,0.,0.));
#9062=DIRECTION('',(0.,0.,-1.));
#9063=DIRECTION('center_axis',(0.,0.,1.));
#9064=DIRECTION('ref_axis',(1.,0.,0.));
#9065=DIRECTION('center_axis',(0.,0.,1.));
#9066=DIRECTION('ref_axis',(1.,0.,0.));
#9067=DIRECTION('',(0.,0.,-1.));
#9068=DIRECTION('center_axis',(0.,0.,1.));
#9069=DIRECTION('ref_axis',(1.,0.,0.));
#9070=DIRECTION('center_axis',(0.,0.,1.));
#9071=DIRECTION('ref_axis',(1.,0.,0.));
#9072=DIRECTION('',(0.,0.,1.));
#9073=DIRECTION('center_axis',(0.,0.,-1.));
#9074=DIRECTION('ref_axis',(-1.,0.,0.));
#9075=DIRECTION('center_axis',(0.,0.,1.));
#9076=DIRECTION('ref_axis',(1.,0.,0.));
#9077=DIRECTION('',(0.,0.,-1.));
#9078=DIRECTION('center_axis',(0.,0.,1.));
#9079=DIRECTION('ref_axis',(1.,0.,0.));
#9080=DIRECTION('center_axis',(0.,0.,1.));
#9081=DIRECTION('ref_axis',(1.,0.,0.));
#9082=DIRECTION('',(0.,0.,1.));
#9083=DIRECTION('center_axis',(0.,0.,-1.));
#9084=DIRECTION('ref_axis',(-1.,0.,0.));
#9085=DIRECTION('center_axis',(0.,0.,1.));
#9086=DIRECTION('ref_axis',(1.,0.,0.));
#9087=DIRECTION('',(0.,0.,-1.));
#9088=DIRECTION('center_axis',(0.,0.,1.));
#9089=DIRECTION('ref_axis',(1.,0.,0.));
#9090=DIRECTION('center_axis',(0.,0.,1.));
#9091=DIRECTION('ref_axis',(1.,0.,0.));
#9092=DIRECTION('',(0.,0.,1.));
#9093=DIRECTION('center_axis',(0.,0.,-1.));
#9094=DIRECTION('ref_axis',(-1.,0.,0.));
#9095=DIRECTION('center_axis',(0.,0.,1.));
#9096=DIRECTION('ref_axis',(1.,0.,0.));
#9097=DIRECTION('',(0.,0.,-1.));
#9098=DIRECTION('center_axis',(0.,0.,1.));
#9099=DIRECTION('ref_axis',(1.,0.,0.));
#9100=DIRECTION('center_axis',(0.,0.,1.));
#9101=DIRECTION('ref_axis',(1.,0.,0.));
#9102=DIRECTION('',(0.,0.,1.));
#9103=DIRECTION('center_axis',(0.,0.,-1.));
#9104=DIRECTION('ref_axis',(-1.,0.,0.));
#9105=DIRECTION('center_axis',(0.,0.,1.));
#9106=DIRECTION('ref_axis',(1.,0.,0.));
#9107=DIRECTION('',(0.,0.,-1.));
#9108=DIRECTION('center_axis',(0.,0.,1.));
#9109=DIRECTION('ref_axis',(1.,0.,0.));
#9110=DIRECTION('center_axis',(0.,0.,1.));
#9111=DIRECTION('ref_axis',(1.,0.,0.));
#9112=DIRECTION('',(0.,0.,1.));
#9113=DIRECTION('center_axis',(0.,0.,-1.));
#9114=DIRECTION('ref_axis',(-1.,0.,0.));
#9115=DIRECTION('center_axis',(0.,0.,1.));
#9116=DIRECTION('ref_axis',(1.,0.,0.));
#9117=DIRECTION('',(0.,0.,-1.));
#9118=DIRECTION('center_axis',(0.,0.,1.));
#9119=DIRECTION('ref_axis',(1.,0.,0.));
#9120=DIRECTION('',(0.,0.,1.));
#9121=DIRECTION('center_axis',(0.,0.,-1.));
#9122=DIRECTION('ref_axis',(-1.,0.,0.));
#9123=DIRECTION('center_axis',(0.,0.,1.));
#9124=DIRECTION('ref_axis',(1.,0.,0.));
#9125=DIRECTION('',(0.,0.,-1.));
#9126=DIRECTION('center_axis',(0.,0.,1.));
#9127=DIRECTION('ref_axis',(1.,0.,0.));
#9128=DIRECTION('',(0.,0.,1.));
#9129=DIRECTION('center_axis',(0.,0.,-1.));
#9130=DIRECTION('ref_axis',(-1.,0.,0.));
#9131=DIRECTION('center_axis',(0.,0.,1.));
#9132=DIRECTION('ref_axis',(1.,0.,0.));
#9133=DIRECTION('',(0.,0.,1.));
#9134=DIRECTION('center_axis',(0.,0.,-1.));
#9135=DIRECTION('ref_axis',(-1.,0.,0.));
#9136=DIRECTION('',(0.,0.,-1.));
#9137=DIRECTION('center_axis',(0.,0.,1.));
#9138=DIRECTION('ref_axis',(1.,0.,0.));
#9139=DIRECTION('center_axis',(0.,0.,1.));
#9140=DIRECTION('ref_axis',(1.,0.,0.));
#9141=DIRECTION('',(0.,0.,1.));
#9142=DIRECTION('center_axis',(0.,0.,-1.));
#9143=DIRECTION('ref_axis',(-1.,0.,0.));
#9144=DIRECTION('',(0.,0.,-1.));
#9145=DIRECTION('center_axis',(0.,0.,1.));
#9146=DIRECTION('ref_axis',(1.,0.,0.));
#9147=DIRECTION('center_axis',(0.,0.,1.));
#9148=DIRECTION('ref_axis',(1.,0.,0.));
#9149=DIRECTION('',(0.,0.,-1.));
#9150=DIRECTION('center_axis',(0.,0.,1.));
#9151=DIRECTION('ref_axis',(1.,0.,0.));
#9152=DIRECTION('',(0.,0.,1.));
#9153=DIRECTION('center_axis',(0.,0.,-1.));
#9154=DIRECTION('ref_axis',(-1.,0.,0.));
#9155=DIRECTION('',(0.,0.,-1.));
#9156=DIRECTION('center_axis',(0.,0.,1.));
#9157=DIRECTION('ref_axis',(1.,0.,0.));
#9158=DIRECTION('',(0.,0.,1.));
#9159=DIRECTION('center_axis',(0.,0.,-1.));
#9160=DIRECTION('ref_axis',(-1.,0.,0.));
#9161=DIRECTION('center_axis',(0.,0.,1.));
#9162=DIRECTION('ref_axis',(1.,0.,0.));
#9163=DIRECTION('',(0.,0.,-1.));
#9164=DIRECTION('center_axis',(0.,0.,1.));
#9165=DIRECTION('ref_axis',(-0.98841174204174,0.15179666726912,0.));
#9166=DIRECTION('',(0.,0.,1.));
#9167=DIRECTION('center_axis',(0.,0.,-1.));
#9168=DIRECTION('ref_axis',(0.802811069346189,-0.596233500346323,0.));
#9169=DIRECTION('',(0.,0.,-1.));
#9170=DIRECTION('center_axis',(0.,0.,1.));
#9171=DIRECTION('ref_axis',(1.,0.,0.));
#9172=DIRECTION('',(0.,0.,1.));
#9173=DIRECTION('center_axis',(0.,0.,-1.));
#9174=DIRECTION('ref_axis',(-1.,0.,0.));
#9175=DIRECTION('center_axis',(0.,0.,1.));
#9176=DIRECTION('ref_axis',(1.,0.,0.));
#9177=DIRECTION('',(0.,0.,-1.));
#9178=DIRECTION('center_axis',(0.,0.,1.));
#9179=DIRECTION('ref_axis',(1.,0.,0.));
#9180=DIRECTION('',(0.,0.,1.));
#9181=DIRECTION('center_axis',(0.,0.,-1.));
#9182=DIRECTION('ref_axis',(0.999945056799679,-0.0104825274569905,0.));
#9183=DIRECTION('',(0.,0.,-1.));
#9184=DIRECTION('center_axis',(0.,0.,1.));
#9185=DIRECTION('ref_axis',(1.,0.,0.));
#9186=DIRECTION('',(0.,0.,1.));
#9187=DIRECTION('center_axis',(0.,0.,-1.));
#9188=DIRECTION('ref_axis',(-1.,0.,0.));
#9189=DIRECTION('center_axis',(0.,0.,1.));
#9190=DIRECTION('ref_axis',(1.,0.,0.));
#9191=DIRECTION('',(0.,0.,-1.));
#9192=DIRECTION('center_axis',(0.,0.,1.));
#9193=DIRECTION('ref_axis',(1.,0.,0.));
#9194=DIRECTION('',(0.,0.,1.));
#9195=DIRECTION('center_axis',(0.,0.,-1.));
#9196=DIRECTION('ref_axis',(0.980273298181861,0.197646808402403,0.));
#9197=DIRECTION('',(0.,0.,-1.));
#9198=DIRECTION('center_axis',(0.,0.,1.));
#9199=DIRECTION('ref_axis',(1.,0.,0.));
#9200=DIRECTION('',(0.,0.,1.));
#9201=DIRECTION('center_axis',(0.,0.,-1.));
#9202=DIRECTION('ref_axis',(-1.,0.,0.));
#9203=DIRECTION('center_axis',(0.,0.,1.));
#9204=DIRECTION('ref_axis',(1.,0.,0.));
#9205=DIRECTION('',(0.,0.,-1.));
#9206=DIRECTION('center_axis',(0.,0.,1.));
#9207=DIRECTION('ref_axis',(1.,0.,0.));
#9208=DIRECTION('',(0.,0.,1.));
#9209=DIRECTION('center_axis',(0.,0.,-1.));
#9210=DIRECTION('ref_axis',(0.975914418166608,-0.218153726565764,0.));
#9211=DIRECTION('',(0.,0.,-1.));
#9212=DIRECTION('center_axis',(0.,0.,1.));
#9213=DIRECTION('ref_axis',(1.,0.,0.));
#9214=DIRECTION('',(0.,0.,1.));
#9215=DIRECTION('center_axis',(0.,0.,-1.));
#9216=DIRECTION('ref_axis',(-1.,0.,0.));
#9217=DIRECTION('center_axis',(0.,0.,1.));
#9218=DIRECTION('ref_axis',(1.,0.,0.));
#9219=DIRECTION('',(0.,0.,-1.));
#9220=DIRECTION('center_axis',(0.,0.,1.));
#9221=DIRECTION('ref_axis',(-0.998372875767673,-0.0570228106233482,0.));
#9222=DIRECTION('',(0.,0.,1.));
#9223=DIRECTION('center_axis',(0.,0.,-1.));
#9224=DIRECTION('ref_axis',(0.909231636502712,-0.416290561005893,0.));
#9225=DIRECTION('',(0.,0.,-1.));
#9226=DIRECTION('center_axis',(0.,0.,1.));
#9227=DIRECTION('ref_axis',(1.,0.,0.));
#9228=DIRECTION('',(0.,0.,1.));
#9229=DIRECTION('center_axis',(0.,0.,-1.));
#9230=DIRECTION('ref_axis',(-1.,0.,0.));
#9231=DIRECTION('center_axis',(0.,0.,1.));
#9232=DIRECTION('ref_axis',(1.,0.,0.));
#9233=DIRECTION('',(0.,0.,-1.));
#9234=DIRECTION('center_axis',(0.,0.,1.));
#9235=DIRECTION('ref_axis',(1.,0.,0.));
#9236=DIRECTION('',(0.,0.,1.));
#9237=DIRECTION('center_axis',(0.,0.,-1.));
#9238=DIRECTION('ref_axis',(0.917758892560324,0.397138030319997,0.));
#9239=DIRECTION('',(0.,0.,-1.));
#9240=DIRECTION('center_axis',(0.,0.,1.));
#9241=DIRECTION('ref_axis',(1.,0.,0.));
#9242=DIRECTION('',(0.,0.,1.));
#9243=DIRECTION('center_axis',(0.,0.,-1.));
#9244=DIRECTION('ref_axis',(-1.,0.,0.));
#9245=DIRECTION('center_axis',(0.,0.,1.));
#9246=DIRECTION('ref_axis',(1.,0.,0.));
#9247=DIRECTION('',(0.,0.,-1.));
#9248=DIRECTION('center_axis',(0.,0.,1.));
#9249=DIRECTION('ref_axis',(1.,0.,0.));
#9250=DIRECTION('',(0.,0.,1.));
#9251=DIRECTION('center_axis',(0.,0.,-1.));
#9252=DIRECTION('ref_axis',(0.815134019438135,0.579272414632899,0.));
#9253=DIRECTION('',(0.,0.,-1.));
#9254=DIRECTION('center_axis',(0.,0.,1.));
#9255=DIRECTION('ref_axis',(1.,0.,0.));
#9256=DIRECTION('',(0.,0.,1.));
#9257=DIRECTION('center_axis',(0.,0.,-1.));
#9258=DIRECTION('ref_axis',(-1.,0.,0.));
#9259=DIRECTION('center_axis',(0.,0.,1.));
#9260=DIRECTION('ref_axis',(1.,0.,0.));
#9261=DIRECTION('',(0.,0.,-1.));
#9262=DIRECTION('center_axis',(0.,0.,1.));
#9263=DIRECTION('ref_axis',(1.,0.,0.));
#9264=DIRECTION('',(0.,0.,1.));
#9265=DIRECTION('center_axis',(0.,0.,-1.));
#9266=DIRECTION('ref_axis',(-1.,0.,0.));
#9267=DIRECTION('',(0.,0.,-1.));
#9268=DIRECTION('center_axis',(0.,0.,1.));
#9269=DIRECTION('ref_axis',(1.,0.,0.));
#9270=DIRECTION('',(0.,0.,1.));
#9271=DIRECTION('center_axis',(0.,0.,-1.));
#9272=DIRECTION('ref_axis',(0.815134019438126,-0.579272414632913,0.));
#9273=DIRECTION('center_axis',(0.,0.,1.));
#9274=DIRECTION('ref_axis',(1.,0.,0.));
#9275=DIRECTION('',(0.,0.,-1.));
#9276=DIRECTION('center_axis',(0.,0.,1.));
#9277=DIRECTION('ref_axis',(1.,0.,0.));
#9278=DIRECTION('',(0.,0.,1.));
#9279=DIRECTION('center_axis',(0.,0.,-1.));
#9280=DIRECTION('ref_axis',(-1.,0.,0.));
#9281=DIRECTION('',(0.,0.,-1.));
#9282=DIRECTION('center_axis',(0.,0.,1.));
#9283=DIRECTION('ref_axis',(1.,0.,0.));
#9284=DIRECTION('',(0.,0.,1.));
#9285=DIRECTION('center_axis',(0.,0.,-1.));
#9286=DIRECTION('ref_axis',(0.91775889256032,-0.397138030320008,0.));
#9287=DIRECTION('center_axis',(0.,0.,1.));
#9288=DIRECTION('ref_axis',(-0.998372875767673,0.0570228106233547,0.));
#9289=DIRECTION('',(0.,0.,-1.));
#9290=DIRECTION('center_axis',(0.,0.,1.));
#9291=DIRECTION('ref_axis',(1.,0.,0.));
#9292=DIRECTION('',(0.,0.,1.));
#9293=DIRECTION('center_axis',(0.,0.,-1.));
#9294=DIRECTION('ref_axis',(-1.,0.,0.));
#9295=DIRECTION('',(0.,0.,-1.));
#9296=DIRECTION('center_axis',(0.,0.,1.));
#9297=DIRECTION('ref_axis',(1.,0.,0.));
#9298=DIRECTION('',(0.,0.,1.));
#9299=DIRECTION('center_axis',(0.,0.,-1.));
#9300=DIRECTION('ref_axis',(0.909231636502715,0.416290561005885,0.));
#9301=DIRECTION('center_axis',(0.,0.,1.));
#9302=DIRECTION('ref_axis',(1.,0.,0.));
#9303=DIRECTION('',(0.,0.,-1.));
#9304=DIRECTION('center_axis',(0.,0.,1.));
#9305=DIRECTION('ref_axis',(1.,0.,0.));
#9306=DIRECTION('',(0.,0.,1.));
#9307=DIRECTION('center_axis',(0.,0.,-1.));
#9308=DIRECTION('ref_axis',(-1.,0.,0.));
#9309=DIRECTION('',(0.,0.,-1.));
#9310=DIRECTION('center_axis',(0.,0.,1.));
#9311=DIRECTION('ref_axis',(1.,0.,0.));
#9312=DIRECTION('',(0.,0.,1.));
#9313=DIRECTION('center_axis',(0.,0.,-1.));
#9314=DIRECTION('ref_axis',(0.975914418166611,0.218153726565752,0.));
#9315=DIRECTION('center_axis',(0.,0.,1.));
#9316=DIRECTION('ref_axis',(1.,0.,0.));
#9317=DIRECTION('',(0.,0.,-1.));
#9318=DIRECTION('center_axis',(0.,0.,1.));
#9319=DIRECTION('ref_axis',(1.,0.,0.));
#9320=DIRECTION('',(0.,0.,1.));
#9321=DIRECTION('center_axis',(0.,0.,-1.));
#9322=DIRECTION('ref_axis',(-1.,0.,0.));
#9323=DIRECTION('',(0.,0.,-1.));
#9324=DIRECTION('center_axis',(0.,0.,1.));
#9325=DIRECTION('ref_axis',(1.,0.,0.));
#9326=DIRECTION('',(0.,0.,1.));
#9327=DIRECTION('center_axis',(0.,0.,-1.));
#9328=DIRECTION('ref_axis',(0.98027329818186,-0.197646808402409,0.));
#9329=DIRECTION('center_axis',(0.,0.,1.));
#9330=DIRECTION('ref_axis',(1.,0.,0.));
#9331=DIRECTION('',(0.,0.,-1.));
#9332=DIRECTION('center_axis',(0.,0.,1.));
#9333=DIRECTION('ref_axis',(1.,0.,0.));
#9334=DIRECTION('',(0.,0.,1.));
#9335=DIRECTION('center_axis',(0.,0.,-1.));
#9336=DIRECTION('ref_axis',(-1.,0.,0.));
#9337=DIRECTION('',(0.,0.,-1.));
#9338=DIRECTION('center_axis',(0.,0.,1.));
#9339=DIRECTION('ref_axis',(1.,0.,0.));
#9340=DIRECTION('',(0.,0.,1.));
#9341=DIRECTION('center_axis',(0.,0.,-1.));
#9342=DIRECTION('ref_axis',(0.999945056799679,0.0104825274569784,0.));
#9343=DIRECTION('center_axis',(-1.,0.,0.));
#9344=DIRECTION('ref_axis',(0.,0.,1.));
#9345=DIRECTION('',(0.,0.,1.));
#9346=DIRECTION('center_axis',(0.,1.,0.));
#9347=DIRECTION('ref_axis',(0.,0.,1.));
#9348=DIRECTION('',(0.,0.,1.));
#9349=DIRECTION('center_axis',(1.,0.,0.));
#9350=DIRECTION('ref_axis',(0.,0.,-1.));
#10298=CARTESIAN_POINT('',(0.,0.,0.));
#10299=CARTESIAN_POINT('Origin',(1.58293517182884E-14,-0.0809177714881197,
-0.999999999999996));
#10300=CARTESIAN_POINT('',(-0.749999999999984,2.82381973816744,-0.999999999999996));
#10301=CARTESIAN_POINT('',(0.750000000000016,2.82381973816744,-0.999999999999996));
#10302=CARTESIAN_POINT('Origin',(1.56865040007378E-14,-0.0809177714881158,
-0.999999999999996));
#10303=CARTESIAN_POINT('',(-0.749999999999984,2.82381973816744,1.));
#10304=CARTESIAN_POINT('',(-0.749999999999984,2.82381973816744,-0.999999999999996));
#10305=CARTESIAN_POINT('',(0.750000000000016,2.82381973816744,1.));
#10306=CARTESIAN_POINT('Origin',(1.56865040007378E-14,-0.0809177714881158,
1.));
#10307=CARTESIAN_POINT('',(0.750000000000016,2.82381973816744,-0.999999999999996));
#10308=CARTESIAN_POINT('Origin',(2.39698905616068,12.3348169415543,-0.999999999999996));
#10309=CARTESIAN_POINT('',(2.34580779517504,12.0697122857598,1.));
#10310=CARTESIAN_POINT('',(2.12840559486948,12.3624380262694,1.));
#10311=CARTESIAN_POINT('Origin',(2.39698905616068,12.3348169415543,1.));
#10312=CARTESIAN_POINT('',(2.34580779517504,12.0697122857598,-0.999999999999996));
#10313=CARTESIAN_POINT('',(2.34580779517504,12.0697122857598,-0.999999999999996));
#10314=CARTESIAN_POINT('',(2.12840559486948,12.3624380262694,-0.999999999999996));
#10315=CARTESIAN_POINT('Origin',(2.39698905616068,12.3348169415543,-0.999999999999996));
#10316=CARTESIAN_POINT('',(2.12840559486948,12.3624380262694,-0.999999999999996));
#10317=CARTESIAN_POINT('Origin',(-1.53976292115091,12.7396719514087,-0.999999999999996));
#10318=CARTESIAN_POINT('',(1.84616149105017,14.2002477183787,-0.999999999999996));
#10319=CARTESIAN_POINT('Origin',(-1.5397629211509,12.7396719514087,-0.999999999999996));
#10320=CARTESIAN_POINT('',(1.84616149105017,14.2002477183787,1.));
#10321=CARTESIAN_POINT('',(1.84616149105017,14.2002477183787,4.11429224827654E-15));
#10322=CARTESIAN_POINT('Origin',(-1.53976292115089,12.7396719514087,1.));
#10323=CARTESIAN_POINT('Origin',(4.92598549120215,11.5651413018837,-0.999999999999996));
#10324=CARTESIAN_POINT('',(4.82080430633663,11.3164710013847,1.));
#10325=CARTESIAN_POINT('',(4.66901396936873,11.6480004411902,1.));
#10326=CARTESIAN_POINT('Origin',(4.92598549120215,11.5651413018837,1.));
#10327=CARTESIAN_POINT('',(4.82080430633663,11.3164710013847,-0.999999999999996));
#10328=CARTESIAN_POINT('',(4.82080430633663,11.3164710013847,-0.999999999999996));
#10329=CARTESIAN_POINT('',(4.66901396936873,11.6480004411902,-0.999999999999996));
#10330=CARTESIAN_POINT('Origin',(4.92598549120215,11.5651413018837,-0.999999999999996));
#10331=CARTESIAN_POINT('',(4.66901396936873,11.6480004411902,-0.999999999999996));
#10332=CARTESIAN_POINT('Origin',(1.15943507954564,12.7796460183509,-0.999999999999996));
#10333=CARTESIAN_POINT('',(4.77503969688432,13.5043314309807,-0.999999999999996));
#10334=CARTESIAN_POINT('Origin',(1.15943507954563,12.7796460183509,-0.999999999999996));
#10335=CARTESIAN_POINT('',(4.77503969688432,13.5043314309807,1.));
#10336=CARTESIAN_POINT('',(4.77503969688432,13.5043314309807,4.11429224827654E-15));
#10337=CARTESIAN_POINT('Origin',(1.15943507954562,12.7796460183509,1.));
#10338=CARTESIAN_POINT('Origin',(2.39698905616043,-12.4966524845306,-0.999999999999996));
#10339=CARTESIAN_POINT('',(2.12840559486923,-12.5242735692457,1.));
#10340=CARTESIAN_POINT('',(2.34580779517479,-12.2315478287361,1.));
#10341=CARTESIAN_POINT('Origin',(2.39698905616042,-12.4966524845306,1.));
#10342=CARTESIAN_POINT('',(2.12840559486923,-12.5242735692457,-0.999999999999996));
#10343=CARTESIAN_POINT('',(2.12840559486923,-12.5242735692457,-0.999999999999996));
#10344=CARTESIAN_POINT('',(2.34580779517479,-12.2315478287361,-0.999999999999996));
#10345=CARTESIAN_POINT('Origin',(2.39698905616042,-12.4966524845306,-0.999999999999996));
#10346=CARTESIAN_POINT('',(2.34580779517479,-12.2315478287361,-0.999999999999996));
#10347=CARTESIAN_POINT('Origin',(-1.53976292115116,-12.9015074943849,-0.999999999999996));
#10348=CARTESIAN_POINT('',(1.84616149104988,-14.362083261355,-0.999999999999996));
#10349=CARTESIAN_POINT('Origin',(-1.53976292115115,-12.9015074943849,-1.));
#10350=CARTESIAN_POINT('',(1.84616149104989,-14.362083261355,1.));
#10351=CARTESIAN_POINT('Origin',(-1.53976292115116,-12.9015074943849,1.));
#10352=CARTESIAN_POINT('',(1.84616149104988,-14.362083261355,4.11429224827654E-15));
#10353=CARTESIAN_POINT('Origin',(4.92598549120192,-11.72697684486,-0.999999999999996));
#10354=CARTESIAN_POINT('',(4.66901396936849,-11.8098359841665,1.));
#10355=CARTESIAN_POINT('',(4.8208043063364,-11.478306544361,1.));
#10356=CARTESIAN_POINT('Origin',(4.92598549120192,-11.72697684486,1.));
#10357=CARTESIAN_POINT('',(4.66901396936849,-11.8098359841665,-0.999999999999996));
#10358=CARTESIAN_POINT('',(4.66901396936849,-11.8098359841665,-0.999999999999996));
#10359=CARTESIAN_POINT('',(4.8208043063364,-11.478306544361,-0.999999999999996));
#10360=CARTESIAN_POINT('Origin',(4.92598549120192,-11.72697684486,-0.999999999999996));
#10361=CARTESIAN_POINT('',(4.8208043063364,-11.478306544361,-0.999999999999996));
#10362=CARTESIAN_POINT('Origin',(1.15943507954538,-12.9414815613272,-0.999999999999996));
#10363=CARTESIAN_POINT('',(4.77503969688405,-13.666166973957,-0.999999999999996));
#10364=CARTESIAN_POINT('Origin',(1.15943507954539,-12.9414815613271,-0.999999999999996));
#10365=CARTESIAN_POINT('',(4.77503969688405,-13.666166973957,1.));
#10366=CARTESIAN_POINT('Origin',(1.15943507954538,-12.9414815613272,1.00000000000001));
#10367=CARTESIAN_POINT('',(4.77503969688405,-13.666166973957,4.11429224827654E-15));
#10368=CARTESIAN_POINT('Origin',(9.23699064246663,-8.71654333487287,-0.999999999999996));
#10369=CARTESIAN_POINT('',(9.03593732412188,-8.89675865936711,1.));
#10370=CARTESIAN_POINT('',(9.03975952554564,-8.53215275344828,1.));
#10371=CARTESIAN_POINT('Origin',(9.23699064246663,-8.71654333487287,1.));
#10372=CARTESIAN_POINT('',(9.03593732412188,-8.89675865936711,-0.999999999999996));
#10373=CARTESIAN_POINT('',(9.03593732412188,-8.89675865936711,-0.999999999999996));
#10374=CARTESIAN_POINT('',(9.03975952554564,-8.53215275344828,-0.999999999999996));
#10375=CARTESIAN_POINT('Origin',(9.23699064246663,-8.71654333487287,-0.999999999999996));
#10376=CARTESIAN_POINT('',(9.03975952554564,-8.53215275344828,-0.999999999999996));
#10377=CARTESIAN_POINT('Origin',(7.23969272277696,-10.4483125396915,-0.999999999999996));
#10378=CARTESIAN_POINT('',(7.0055640289916,-10.5827883915994,1.));
#10379=CARTESIAN_POINT('',(7.0851085365255,-10.2269446798722,1.));
#10380=CARTESIAN_POINT('Origin',(7.23969272277696,-10.4483125396915,1.));
#10381=CARTESIAN_POINT('',(7.0055640289916,-10.5827883915994,-0.999999999999996));
#10382=CARTESIAN_POINT('',(7.0055640289916,-10.5827883915994,-0.999999999999996));
#10383=CARTESIAN_POINT('',(7.0851085365255,-10.2269446798722,-0.999999999999996));
#10384=CARTESIAN_POINT('Origin',(7.23969272277696,-10.4483125396915,-0.999999999999996));
#10385=CARTESIAN_POINT('',(7.0851085365255,-10.2269446798722,-0.999999999999996));
#10386=CARTESIAN_POINT('Origin',(10.8305877470817,-6.60735585460537,-0.999999999999996));
#10387=CARTESIAN_POINT('',(10.6713967989501,-6.82543437723646,1.));
#10388=CARTESIAN_POINT('',(10.5993296457206,-6.46800130478792,1.));
#10389=CARTESIAN_POINT('Origin',(10.8305877470817,-6.60735585460537,1.));
#10390=CARTESIAN_POINT('',(10.6713967989501,-6.82543437723646,-0.999999999999996));
#10391=CARTESIAN_POINT('',(10.6713967989501,-6.82543437723646,-0.999999999999996));
#10392=CARTESIAN_POINT('',(10.5993296457206,-6.46800130478792,-0.999999999999996));
#10393=CARTESIAN_POINT('Origin',(10.8305877470817,-6.60735585460537,-0.999999999999995));
#10394=CARTESIAN_POINT('',(10.5993296457206,-6.46800130478792,-0.999999999999996));
#10395=CARTESIAN_POINT('Origin',(11.9508361962233,-4.21293171278112,-0.999999999999996));
#10396=CARTESIAN_POINT('',(11.8404650266211,-4.45934235565321,1.));
#10397=CARTESIAN_POINT('',(11.6956581991509,-4.12470365709515,1.));
#10398=CARTESIAN_POINT('Origin',(11.9508361962233,-4.21293171278112,1.));
#10399=CARTESIAN_POINT('',(11.8404650266211,-4.45934235565321,-0.999999999999996));
#10400=CARTESIAN_POINT('',(11.8404650266211,-4.45934235565321,-0.999999999999996));
#10401=CARTESIAN_POINT('',(11.6956581991509,-4.12470365709515,-0.999999999999996));
#10402=CARTESIAN_POINT('Origin',(11.9508361962233,-4.21293171278112,-0.999999999999996));
#10403=CARTESIAN_POINT('',(11.6956581991509,-4.12470365709515,-0.999999999999996));
#10404=CARTESIAN_POINT('Origin',(12.5487757571153,-1.63791873411964,-0.999999999999996));
#10405=CARTESIAN_POINT('',(12.4920481157737,-1.90189216972978,1.));
#10406=CARTESIAN_POINT('',(12.2808303672837,-1.6046731619638,1.));
#10407=CARTESIAN_POINT('Origin',(12.5487757571153,-1.63791873411964,1.));
#10408=CARTESIAN_POINT('',(12.4920481157737,-1.90189216972978,-0.999999999999996));
#10409=CARTESIAN_POINT('',(12.4920481157737,-1.90189216972978,-0.999999999999996));
#10410=CARTESIAN_POINT('',(12.2808303672837,-1.6046731619638,-0.999999999999996));
#10411=CARTESIAN_POINT('Origin',(12.5487757571153,-1.63791873411964,-0.999999999999996));
#10412=CARTESIAN_POINT('',(12.2808303672837,-1.6046731619638,-0.999999999999996));
#10413=CARTESIAN_POINT('Origin',(12.5487757571153,1.47608319114314,-0.999999999999996));
#10414=CARTESIAN_POINT('',(12.2808303672837,1.44283761898731,1.));
#10415=CARTESIAN_POINT('',(12.4920481157738,1.74005662675329,1.));
#10416=CARTESIAN_POINT('Origin',(12.5487757571153,1.47608319114314,1.));
#10417=CARTESIAN_POINT('',(12.2808303672837,1.44283761898731,-0.999999999999996));
#10418=CARTESIAN_POINT('',(12.2808303672837,1.44283761898731,-0.999999999999996));
#10419=CARTESIAN_POINT('',(12.4920481157738,1.74005662675329,-0.999999999999996));
#10420=CARTESIAN_POINT('Origin',(12.5487757571153,1.47608319114314,-0.999999999999996));
#10421=CARTESIAN_POINT('',(12.4920481157738,1.74005662675329,-0.999999999999996));
#10422=CARTESIAN_POINT('Origin',(9.23699064246681,8.55470779189644,-0.999999999999996));
#10423=CARTESIAN_POINT('',(9.03975952554581,8.37031721047186,1.));
#10424=CARTESIAN_POINT('',(9.03593732412206,8.73492311639068,1.));
#10425=CARTESIAN_POINT('Origin',(9.23699064246681,8.55470779189644,1.));
#10426=CARTESIAN_POINT('',(9.03975952554581,8.37031721047186,-0.999999999999996));
#10427=CARTESIAN_POINT('',(9.03975952554581,8.37031721047186,-0.999999999999996));
#10428=CARTESIAN_POINT('',(9.03593732412206,8.73492311639068,-0.999999999999996));
#10429=CARTESIAN_POINT('Origin',(9.23699064246681,8.55470779189644,-0.999999999999996));
#10430=CARTESIAN_POINT('',(9.03593732412206,8.73492311639068,-0.999999999999996));
#10431=CARTESIAN_POINT('Origin',(7.23969272277717,10.2864769967151,-0.999999999999996));
#10432=CARTESIAN_POINT('',(7.08510853652571,10.0651091368958,1.));
#10433=CARTESIAN_POINT('',(7.00556402899182,10.420952848623,1.));
#10434=CARTESIAN_POINT('Origin',(7.23969272277717,10.2864769967151,1.));
#10435=CARTESIAN_POINT('',(7.08510853652571,10.0651091368958,-0.999999999999996));
#10436=CARTESIAN_POINT('',(7.08510853652571,10.0651091368958,-0.999999999999996));
#10437=CARTESIAN_POINT('',(7.00556402899182,10.420952848623,-0.999999999999996));
#10438=CARTESIAN_POINT('Origin',(7.23969272277717,10.2864769967151,-0.999999999999996));
#10439=CARTESIAN_POINT('',(7.00556402899182,10.420952848623,-0.999999999999996));
#10440=CARTESIAN_POINT('Origin',(10.8305877470819,6.4455203116289,-0.999999999999996));
#10441=CARTESIAN_POINT('',(10.5993296457207,6.30616576181146,1.));
#10442=CARTESIAN_POINT('',(10.6713967989503,6.66359883425999,1.));
#10443=CARTESIAN_POINT('Origin',(10.8305877470819,6.44552031162891,1.));
#10444=CARTESIAN_POINT('',(10.5993296457207,6.30616576181146,-0.999999999999996));
#10445=CARTESIAN_POINT('',(10.5993296457207,6.30616576181146,-0.999999999999996));
#10446=CARTESIAN_POINT('',(10.6713967989503,6.66359883425999,-0.999999999999996));
#10447=CARTESIAN_POINT('Origin',(10.8305877470819,6.44552031162891,-0.999999999999995));
#10448=CARTESIAN_POINT('',(10.6713967989503,6.66359883425999,-0.999999999999996));
#10449=CARTESIAN_POINT('Origin',(11.9508361962234,4.05109616980463,-0.999999999999996));
#10450=CARTESIAN_POINT('',(11.695658199151,3.96286811411867,1.));
#10451=CARTESIAN_POINT('',(11.8404650266212,4.29750681267673,1.));
#10452=CARTESIAN_POINT('Origin',(11.9508361962234,4.05109616980463,1.));
#10453=CARTESIAN_POINT('',(11.695658199151,3.96286811411867,-0.999999999999996));
#10454=CARTESIAN_POINT('',(11.695658199151,3.96286811411867,-0.999999999999996));
#10455=CARTESIAN_POINT('',(11.8404650266212,4.29750681267673,-0.999999999999996));
#10456=CARTESIAN_POINT('Origin',(11.9508361962234,4.05109616980463,-0.999999999999996));
#10457=CARTESIAN_POINT('',(11.8404650266212,4.29750681267673,-0.999999999999996));
#10458=CARTESIAN_POINT('Origin',(1.56125112837913E-14,-0.080917771488119,
1.));
#10459=CARTESIAN_POINT('',(-14.3959081946537,0.26234197142012,1.));
#10460=CARTESIAN_POINT('',(-14.3959081946537,-0.424177514396259,1.));
#10461=CARTESIAN_POINT('Origin',(-1.64885466391596E-12,-0.0809177714880671,
1.00000000000058));
#10462=CARTESIAN_POINT('',(-14.3959081946537,0.262341971420116,-0.999999999999996));
#10463=CARTESIAN_POINT('',(-14.3959081946537,0.262341971420116,4.11429224827654E-15));
#10464=CARTESIAN_POINT('',(-14.3959081946537,-0.424177514396258,-0.999999999999996));
#10465=CARTESIAN_POINT('Origin',(-1.91426735574041E-12,-0.0809177714880703,
-1.00000000000057));
#10466=CARTESIAN_POINT('',(-14.3959081946537,-0.424177514396259,4.11429224827654E-15));
#10467=CARTESIAN_POINT('Origin',(1.56125112837913E-14,-0.080917771488119,
1.));
#10468=CARTESIAN_POINT('',(-9.88783448111204,-10.5494768544819,1.));
#10469=CARTESIAN_POINT('',(-9.37765107763819,-11.0088480543034,1.));
#10470=CARTESIAN_POINT('Origin',(-6.10622663543836E-13,-0.0809177714888648,
1.00000000000058));
#10471=CARTESIAN_POINT('',(-9.88783448111203,-10.5494768544819,-0.999999999999996));
#10472=CARTESIAN_POINT('',(-9.88783448111203,-10.5494768544819,4.11429224827654E-15));
#10473=CARTESIAN_POINT('',(-9.37765107763819,-11.0088480543034,-0.999999999999996));
#10474=CARTESIAN_POINT('Origin',(2.08166817117217E-13,-0.0809177714878881,
-1.00000000000057));
#10475=CARTESIAN_POINT('',(-9.37765107763819,-11.0088480543034,4.11429224827654E-15));
#10476=CARTESIAN_POINT('Origin',(1.56125112837913E-14,-0.080917771488119,
1.));
#10477=CARTESIAN_POINT('',(-11.8482973935236,-8.26491733616443,-0.999999999999996));
#10478=CARTESIAN_POINT('',(-11.4447713643493,-8.82032326715943,-0.999999999999996));
#10479=CARTESIAN_POINT('Origin',(3.06005221162309E-12,-0.0809177714858984,
-1.00000000000057));
#10480=CARTESIAN_POINT('',(-11.4447713643493,-8.82032326715942,1.));
#10481=CARTESIAN_POINT('',(-11.4447713643493,-8.82032326715943,4.11429224827654E-15));
#10482=CARTESIAN_POINT('',(-11.8482973935236,-8.26491733616442,1.));
#10483=CARTESIAN_POINT('Origin',(1.35221694952392E-12,-0.0809177714871127,
1.00000000000058));
#10484=CARTESIAN_POINT('',(-11.8482973935236,-8.26491733616443,4.11429224827654E-15));
#10485=CARTESIAN_POINT('Origin',(1.56125112837913E-14,-0.080917771488119,
1.));
#10486=CARTESIAN_POINT('',(-7.49522575478187,-12.3765101071527,1.));
#10487=CARTESIAN_POINT('',(-6.90068243987186,-12.7197698500609,1.));
#10488=CARTESIAN_POINT('Origin',(3.30031141304588E-13,-0.0809177714875715,
1.00000000000058));
#10489=CARTESIAN_POINT('',(-7.49522575478187,-12.3765101071527,-0.999999999999996));
#10490=CARTESIAN_POINT('',(-7.49522575478187,-12.3765101071527,4.11429224827654E-15));
#10491=CARTESIAN_POINT('',(-6.90068243987186,-12.7197698500609,-0.999999999999996));
#10492=CARTESIAN_POINT('Origin',(3.30031141304588E-13,-0.0809177714875715,
-1.00000000000057));
#10493=CARTESIAN_POINT('',(-6.90068243987186,-12.7197698500609,4.11429224827654E-15));
#10494=CARTESIAN_POINT('Origin',(1.56125112837913E-14,-0.080917771488119,
1.));
#10495=CARTESIAN_POINT('',(-4.7750396968842,-13.666166973957,1.));
#10496=CARTESIAN_POINT('',(-4.12212086633492,-13.8783131620438,1.));
#10497=CARTESIAN_POINT('Origin',(-7.39859562504108E-13,-0.0809177714905249,
1.00000000000058));
#10498=CARTESIAN_POINT('',(-4.7750396968842,-13.666166973957,-0.999999999999996));
#10499=CARTESIAN_POINT('',(-4.7750396968842,-13.666166973957,4.11429224827654E-15));
#10500=CARTESIAN_POINT('',(-4.12212086633494,-13.8783131620438,-0.999999999999996));
#10501=CARTESIAN_POINT('Origin',(5.34294830600857E-13,-0.0809177714868057,
-1.00000000000057));
#10502=CARTESIAN_POINT('',(-4.12212086633494,-13.8783131620438,4.11429224827654E-15));
#10503=CARTESIAN_POINT('Origin',(1.56125112837913E-14,-0.080917771488119,
1.));
#10504=CARTESIAN_POINT('',(-13.2909328553994,-5.62267776568361,-0.999999999999996));
#10505=CARTESIAN_POINT('',(-13.0117002243323,-6.24984452353429,-0.999999999999996));
#10506=CARTESIAN_POINT('Origin',(-2.78076173199082E-12,-0.0809177714893193,
-1.00000000000057));
#10507=CARTESIAN_POINT('',(-13.0117002243323,-6.24984452353429,1.));
#10508=CARTESIAN_POINT('',(-13.0117002243323,-6.24984452353429,4.11429224827654E-15));
#10509=CARTESIAN_POINT('',(-13.2909328553994,-5.62267776568361,1.));
#10510=CARTESIAN_POINT('Origin',(-2.78076173199082E-12,-0.0809177714893193,
1.00000000000058));
#10511=CARTESIAN_POINT('',(-13.2909328553994,-5.62267776568361,4.11429224827654E-15));
#10512=CARTESIAN_POINT('Origin',(1.56125112837913E-14,-0.080917771488119,
1.));
#10513=CARTESIAN_POINT('',(-14.1526907745224,-2.73823669114163,-0.999999999999996));
#10514=CARTESIAN_POINT('',(-14.009955347447,-3.40975407904992,-0.999999999999996));
#10515=CARTESIAN_POINT('Origin',(2.91433543964104E-13,-0.0809177714879744,
-1.00000000000057));
#10516=CARTESIAN_POINT('',(-14.009955347447,-3.40975407904993,1.));
#10517=CARTESIAN_POINT('',(-14.009955347447,-3.40975407904992,4.11429224827654E-15));
#10518=CARTESIAN_POINT('',(-14.1526907745224,-2.73823669114163,1.));
#10519=CARTESIAN_POINT('Origin',(-1.5256892971216E-12,-0.0809177714883608,
1.00000000000058));
#10520=CARTESIAN_POINT('',(-14.1526907745224,-2.73823669114163,4.11429224827654E-15));
#10521=CARTESIAN_POINT('Origin',(1.56125112837913E-14,-0.080917771488119,
1.));
#10522=CARTESIAN_POINT('',(-14.0099553474469,3.24791853607378,-0.999999999999996));
#10523=CARTESIAN_POINT('',(-14.1526907745224,2.57640114816549,-0.999999999999996));
#10524=CARTESIAN_POINT('Origin',(6.50521303491303E-14,-0.0809177714881221,
-1.00000000000057));
#10525=CARTESIAN_POINT('',(-14.1526907745224,2.57640114816548,1.));
#10526=CARTESIAN_POINT('',(-14.1526907745224,2.57640114816548,4.11429224827654E-15));
#10527=CARTESIAN_POINT('',(-14.0099553474469,3.24791853607378,1.));
#10528=CARTESIAN_POINT('Origin',(3.01841884819964E-13,-0.080917771488147,
1.00000000000058));
#10529=CARTESIAN_POINT('',(-14.0099553474469,3.24791853607378,4.11429224827654E-15));
#10530=CARTESIAN_POINT('Origin',(1.56125112837913E-14,-0.080917771488119,
1.));
#10531=CARTESIAN_POINT('',(-6.90068243987177,12.5579343070847,1.));
#10532=CARTESIAN_POINT('',(-7.49522575478179,12.2146745641765,1.));
#10533=CARTESIAN_POINT('Origin',(8.31799906730879E-13,-0.0809177714895326,
1.00000000000058));
#10534=CARTESIAN_POINT('',(-6.90068243987177,12.5579343070847,-0.999999999999996));
#10535=CARTESIAN_POINT('',(-6.90068243987177,12.5579343070847,4.11429224827654E-15));
#10536=CARTESIAN_POINT('',(-7.49522575478179,12.2146745641765,-0.999999999999996));
#10537=CARTESIAN_POINT('Origin',(8.31799906730879E-13,-0.0809177714895326,
-1.00000000000057));
#10538=CARTESIAN_POINT('',(-7.49522575478179,12.2146745641765,4.11429224827654E-15));
#10539=CARTESIAN_POINT('Origin',(1.56125112837913E-14,-0.080917771488119,
1.));
#10540=CARTESIAN_POINT('',(-9.37765107763812,10.8470125113272,1.));
#10541=CARTESIAN_POINT('',(-9.88783448111196,10.3876413115057,1.));
#10542=CARTESIAN_POINT('Origin',(3.41740524767431E-13,-0.0809177714884615,
1.00000000000058));
#10543=CARTESIAN_POINT('',(-9.37765107763812,10.8470125113272,-0.999999999999996));
#10544=CARTESIAN_POINT('',(-9.37765107763812,10.8470125113272,4.11429224827654E-15));
#10545=CARTESIAN_POINT('',(-9.88783448111196,10.3876413115057,-0.999999999999996));
#10546=CARTESIAN_POINT('Origin',(1.16226472890446E-13,-0.0809177714881162,
-1.00000000000057));
#10547=CARTESIAN_POINT('',(-9.88783448111196,10.3876413115057,4.11429224827654E-15));
#10548=CARTESIAN_POINT('Origin',(1.56125112837913E-14,-0.080917771488119,
1.));
#10549=CARTESIAN_POINT('',(-13.0117002243322,6.08800898055815,-0.999999999999996));
#10550=CARTESIAN_POINT('',(-13.2909328553993,5.46084222270746,-0.999999999999996));
#10551=CARTESIAN_POINT('Origin',(-7.91033905045424E-13,-0.0809177714877533,
-1.00000000000057));
#10552=CARTESIAN_POINT('',(-13.2909328553993,5.46084222270746,1.));
#10553=CARTESIAN_POINT('',(-13.2909328553993,5.46084222270746,4.11429224827654E-15));
#10554=CARTESIAN_POINT('',(-13.0117002243322,6.08800898055815,1.));
#10555=CARTESIAN_POINT('Origin',(-5.57713597526543E-13,-0.0809177714879142,
1.00000000000058));
#10556=CARTESIAN_POINT('',(-13.0117002243322,6.08800898055815,4.11429224827654E-15));
#10557=CARTESIAN_POINT('Origin',(1.56125112837913E-14,-0.080917771488119,
1.));
#10558=CARTESIAN_POINT('',(-11.4447713643492,8.65848772418326,-0.999999999999996));
#10559=CARTESIAN_POINT('',(-11.8482973935235,8.10308179318827,-0.999999999999996));
#10560=CARTESIAN_POINT('Origin',(-9.2374025095765E-13,-0.0809177714874276,
-1.00000000000057));
#10561=CARTESIAN_POINT('',(-11.8482973935235,8.10308179318827,1.));
#10562=CARTESIAN_POINT('',(-11.8482973935235,8.10308179318827,4.11429224827654E-15));
#10563=CARTESIAN_POINT('',(-11.4447713643492,8.65848772418327,1.));
#10564=CARTESIAN_POINT('Origin',(-9.2374025095765E-13,-0.0809177714874276,
1.00000000000058));
#10565=CARTESIAN_POINT('',(-11.4447713643492,8.65848772418326,4.11429224827654E-15));
#10566=CARTESIAN_POINT('Origin',(1.56125112837913E-14,-0.080917771488119,
1.));
#10567=CARTESIAN_POINT('',(-4.12212086633484,13.7164776190675,-0.999999999999996));
#10568=CARTESIAN_POINT('',(-4.7750396968841,13.5043314309807,-0.999999999999996));
#10569=CARTESIAN_POINT('Origin',(5.96311194867027E-13,-0.0809177714895457,
-1.00000000000057));
#10570=CARTESIAN_POINT('',(-4.7750396968841,13.5043314309807,1.));
#10571=CARTESIAN_POINT('',(-4.7750396968841,13.5043314309807,4.11429224827654E-15));
#10572=CARTESIAN_POINT('',(-4.12212086633484,13.7164776190676,1.));
#10573=CARTESIAN_POINT('Origin',(5.23886489744996E-13,-0.0809177714893947,
1.00000000000058));
#10574=CARTESIAN_POINT('',(-4.12212086633484,13.7164776190675,4.11429224827654E-15));
#10575=CARTESIAN_POINT('Origin',(1.56125112837913E-14,-0.080917771488119,
1.));
#10576=CARTESIAN_POINT('',(-1.16340283080869,14.2720085452344,-0.999999999999996));
#10577=CARTESIAN_POINT('',(-1.84616149104994,14.2002477183787,-0.999999999999996));
#10578=CARTESIAN_POINT('Origin',(4.23489368572838E-13,-0.0809177714917566,
-1.00000000000057));
#10579=CARTESIAN_POINT('',(-1.84616149104994,14.2002477183787,1.));
#10580=CARTESIAN_POINT('',(-1.84616149104994,14.2002477183787,4.11429224827654E-15));
#10581=CARTESIAN_POINT('',(-1.16340283080868,14.2720085452344,1.));
#10582=CARTESIAN_POINT('Origin',(4.41378704418849E-13,-0.0809177714920367,
1.00000000000058));
#10583=CARTESIAN_POINT('',(-1.16340283080869,14.2720085452344,4.11429224827654E-15));
#10584=CARTESIAN_POINT('Origin',(1.56125112837913E-14,-0.080917771488119,
1.));
#10585=CARTESIAN_POINT('',(1.16340283080872,14.2720085452344,-0.999999999999996));
#10586=CARTESIAN_POINT('Origin',(-1.63714528045311E-14,-0.0809177714885716,
-1.00000000000057));
#10587=CARTESIAN_POINT('',(1.16340283080872,14.2720085452344,1.));
#10588=CARTESIAN_POINT('',(1.16340283080872,14.2720085452344,4.11429224827654E-15));
#10589=CARTESIAN_POINT('Origin',(-2.37440275774325E-14,-0.0809177714887312,
1.00000000000058));
#10590=CARTESIAN_POINT('Origin',(1.56125112837913E-14,-0.080917771488119,
1.));
#10591=CARTESIAN_POINT('',(4.12212086633506,13.7164776190675,-0.999999999999996));
#10592=CARTESIAN_POINT('Origin',(2.3115190317391E-13,-0.0809177714871977,
-1.00000000000057));
#10593=CARTESIAN_POINT('',(4.12212086633506,13.7164776190675,1.));
#10594=CARTESIAN_POINT('',(4.12212086633506,13.7164776190675,4.11429224827654E-15));
#10595=CARTESIAN_POINT('Origin',(9.15066633577766E-14,-0.0809177714876609,
1.00000000000058));
#10596=CARTESIAN_POINT('Origin',(1.56125112837913E-14,-0.080917771488119,
1.));
#10597=CARTESIAN_POINT('',(4.12212086633478,-13.8783131620438,1.));
#10598=CARTESIAN_POINT('Origin',(-4.75747913286639E-13,-0.0809177714867961,
1.00000000000058));
#10599=CARTESIAN_POINT('',(4.12212086633479,-13.8783131620438,-0.999999999999996));
#10600=CARTESIAN_POINT('',(4.12212086633479,-13.8783131620438,4.11429224827654E-15));
#10601=CARTESIAN_POINT('Origin',(-4.75747913286639E-13,-0.0809177714867961,
-1.00000000000057));
#10602=CARTESIAN_POINT('Origin',(1.56125112837913E-14,-0.080917771488119,
1.));
#10603=CARTESIAN_POINT('',(6.90068243987172,-12.719769850061,1.));
#10604=CARTESIAN_POINT('',(7.49522575478174,-12.3765101071528,1.));
#10605=CARTESIAN_POINT('Origin',(-1.02955838299224E-12,-0.0809177714864821,
1.00000000000058));
#10606=CARTESIAN_POINT('',(6.90068243987173,-12.719769850061,-0.999999999999996));
#10607=CARTESIAN_POINT('',(6.90068243987173,-12.719769850061,4.11429224827654E-15));
#10608=CARTESIAN_POINT('',(7.49522575478174,-12.3765101071528,-0.999999999999996));
#10609=CARTESIAN_POINT('Origin',(-3.17020715234761E-13,-0.0809177714876869,
-1.00000000000057));
#10610=CARTESIAN_POINT('',(7.49522575478174,-12.3765101071528,4.11429224827654E-15));
#10611=CARTESIAN_POINT('Origin',(1.56125112837913E-14,-0.080917771488119,
1.));
#10612=CARTESIAN_POINT('',(11.4447713643492,-8.82032326715959,1.));
#10613=CARTESIAN_POINT('',(11.8482973935235,-8.26491733616459,1.));
#10614=CARTESIAN_POINT('Origin',(-6.05418493115906E-13,-0.0809177714877095,
1.00000000000058));
#10615=CARTESIAN_POINT('',(11.4447713643492,-8.82032326715958,-0.999999999999996));
#10616=CARTESIAN_POINT('',(11.4447713643492,-8.82032326715958,4.11429224827654E-15));
#10617=CARTESIAN_POINT('',(11.8482973935235,-8.26491733616459,-0.999999999999996));
#10618=CARTESIAN_POINT('Origin',(-8.26595736302949E-13,-0.0809177714874432,
-1.00000000000057));
#10619=CARTESIAN_POINT('',(11.8482973935235,-8.26491733616459,4.11429224827654E-15));
#10620=CARTESIAN_POINT('Origin',(1.56125112837913E-14,-0.080917771488119,
1.));
#10621=CARTESIAN_POINT('',(9.37765107763808,-11.0088480543035,-0.999999999999996));
#10622=CARTESIAN_POINT('',(9.88783448111192,-10.549476854482,-0.999999999999996));
#10623=CARTESIAN_POINT('Origin',(-2.78423117894278E-13,-0.0809177714878413,
-1.00000000000057));
#10624=CARTESIAN_POINT('',(9.88783448111192,-10.549476854482,1.));
#10625=CARTESIAN_POINT('',(9.88783448111192,-10.549476854482,4.11429224827654E-15));
#10626=CARTESIAN_POINT('',(9.37765107763808,-11.0088480543035,1.));
#10627=CARTESIAN_POINT('Origin',(-2.78423117894278E-13,-0.0809177714878413,
1.00000000000058));
#10628=CARTESIAN_POINT('',(9.37765107763808,-11.0088480543035,4.11429224827654E-15));
#10629=CARTESIAN_POINT('Origin',(1.56125112837913E-14,-0.080917771488119,
1.));
#10630=CARTESIAN_POINT('',(13.0117002243322,-6.24984452353448,1.));
#10631=CARTESIAN_POINT('',(13.2909328553993,-5.62267776568378,1.));
#10632=CARTESIAN_POINT('Origin',(3.37403716077489E-13,-0.0809177714882576,
1.00000000000058));
#10633=CARTESIAN_POINT('',(13.0117002243322,-6.24984452353447,-0.999999999999996));
#10634=CARTESIAN_POINT('',(13.0117002243322,-6.24984452353448,4.11429224827654E-15));
#10635=CARTESIAN_POINT('',(13.2909328553993,-5.62267776568379,-0.999999999999996));
#10636=CARTESIAN_POINT('Origin',(3.37403716077489E-13,-0.0809177714882576,
-1.00000000000057));
#10637=CARTESIAN_POINT('',(13.2909328553993,-5.62267776568379,4.11429224827654E-15));
#10638=CARTESIAN_POINT('Origin',(1.56125112837913E-14,-0.080917771488119,
1.));
#10639=CARTESIAN_POINT('',(14.009955347447,-3.40975407905011,1.));
#10640=CARTESIAN_POINT('',(14.1526907745224,-2.73823669114181,1.));
#10641=CARTESIAN_POINT('Origin',(-2.28549817959944E-12,-0.0809177714875657,
1.00000000000058));
#10642=CARTESIAN_POINT('',(14.009955347447,-3.40975407905011,-0.999999999999996));
#10643=CARTESIAN_POINT('',(14.009955347447,-3.40975407905011,4.11429224827654E-15));
#10644=CARTESIAN_POINT('',(14.1526907745224,-2.73823669114182,-0.999999999999996));
#10645=CARTESIAN_POINT('Origin',(-2.28549817959944E-12,-0.0809177714875657,
-1.00000000000057));
#10646=CARTESIAN_POINT('',(14.1526907745224,-2.73823669114182,4.11429224827654E-15));
#10647=CARTESIAN_POINT('Origin',(1.56125112837913E-14,-0.080917771488119,
1.));
#10648=CARTESIAN_POINT('',(14.3959081946538,-0.424177514396453,1.));
#10649=CARTESIAN_POINT('',(14.3959081946538,0.262341971419921,1.));
#10650=CARTESIAN_POINT('Origin',(1.59681295963665E-12,-0.0809177714880441,
1.00000000000058));
#10651=CARTESIAN_POINT('',(14.3959081946537,-0.42417751439645,-0.999999999999996));
#10652=CARTESIAN_POINT('',(14.3959081946537,-0.42417751439645,4.11429224827654E-15));
#10653=CARTESIAN_POINT('',(14.3959081946538,0.262341971419921,-0.999999999999996));
#10654=CARTESIAN_POINT('Origin',(1.59681295963665E-12,-0.0809177714880441,
-1.00000000000057));
#10655=CARTESIAN_POINT('',(14.3959081946538,0.262341971419922,4.11429224827654E-15));
#10656=CARTESIAN_POINT('Origin',(1.56125112837913E-14,-0.080917771488119,
1.));
#10657=CARTESIAN_POINT('',(14.1526907745224,2.57640114816529,1.));
#10658=CARTESIAN_POINT('',(14.009955347447,3.24791853607358,1.));
#10659=CARTESIAN_POINT('Origin',(-2.38958158815805E-12,-0.0809177714885389,
1.00000000000058));
#10660=CARTESIAN_POINT('',(14.1526907745224,2.57640114816529,-0.999999999999996));
#10661=CARTESIAN_POINT('',(14.1526907745224,2.57640114816529,4.11429224827654E-15));
#10662=CARTESIAN_POINT('',(14.009955347447,3.24791853607358,-0.999999999999996));
#10663=CARTESIAN_POINT('Origin',(1.04083408558608E-14,-0.0809177714880989,
-1.00000000000057));
#10664=CARTESIAN_POINT('',(14.009955347447,3.24791853607358,4.11429224827654E-15));
#10665=CARTESIAN_POINT('Origin',(1.56125112837913E-14,-0.080917771488119,
1.));
#10666=CARTESIAN_POINT('',(9.88783448111214,10.3876413115056,1.));
#10667=CARTESIAN_POINT('',(9.3776510776383,10.8470125113271,1.));
#10668=CARTESIAN_POINT('Origin',(-2.56739074444567E-13,-0.0809177714883591,
1.00000000000058));
#10669=CARTESIAN_POINT('',(9.88783448111214,10.3876413115056,-0.999999999999996));
#10670=CARTESIAN_POINT('',(9.88783448111214,10.3876413115056,4.11429224827654E-15));
#10671=CARTESIAN_POINT('',(9.3776510776383,10.8470125113271,-0.999999999999996));
#10672=CARTESIAN_POINT('Origin',(7.92768628521401E-13,-0.0809177714871318,
-1.00000000000057));
#10673=CARTESIAN_POINT('',(9.3776510776383,10.8470125113271,4.11429224827654E-15));
#10674=CARTESIAN_POINT('Origin',(1.56125112837913E-14,-0.080917771488119,
1.));
#10675=CARTESIAN_POINT('',(7.49522575478199,12.2146745641764,-0.999999999999996));
#10676=CARTESIAN_POINT('',(6.90068243987198,12.5579343070846,-0.999999999999996));
#10677=CARTESIAN_POINT('Origin',(-1.11586087592208E-12,-0.0809177714900123,
-1.00000000000057));
#10678=CARTESIAN_POINT('',(6.90068243987197,12.5579343070846,1.));
#10679=CARTESIAN_POINT('',(6.90068243987198,12.5579343070846,4.11429224827654E-15));
#10680=CARTESIAN_POINT('',(7.49522575478199,12.2146745641764,1.));
#10681=CARTESIAN_POINT('Origin',(-1.04864034122798E-12,-0.0809177714898978,
1.00000000000058));
#10682=CARTESIAN_POINT('',(7.49522575478199,12.2146745641764,4.11429224827654E-15));
#10683=CARTESIAN_POINT('Origin',(1.56125112837913E-14,-0.080917771488119,
1.));
#10684=CARTESIAN_POINT('',(11.8482973935237,8.1030817931881,-0.999999999999996));
#10685=CARTESIAN_POINT('',(11.4447713643494,8.65848772418311,-0.999999999999996));
#10686=CARTESIAN_POINT('Origin',(-2.41386771682173E-12,-0.0809177714898883,
-1.00000000000057));
#10687=CARTESIAN_POINT('',(11.4447713643494,8.65848772418311,1.));
#10688=CARTESIAN_POINT('',(11.4447713643494,8.65848772418311,4.11429224827654E-15));
#10689=CARTESIAN_POINT('',(11.8482973935237,8.1030817931881,1.));
#10690=CARTESIAN_POINT('Origin',(-1.56385321359309E-12,-0.0809177714893453,
1.00000000000058));
#10691=CARTESIAN_POINT('',(11.8482973935237,8.1030817931881,4.11429224827654E-15));
#10692=CARTESIAN_POINT('Origin',(1.56125112837913E-14,-0.080917771488119,
1.));
#10693=CARTESIAN_POINT('',(13.2909328553994,5.46084222270728,-0.999999999999996));
#10694=CARTESIAN_POINT('',(13.0117002243324,6.08800898055796,-0.999999999999996));
#10695=CARTESIAN_POINT('Origin',(1.32879818259823E-12,-0.080917771487513,
-1.00000000000057));
#10696=CARTESIAN_POINT('',(13.0117002243324,6.08800898055796,1.));
#10697=CARTESIAN_POINT('',(13.0117002243324,6.08800898055796,4.11429224827654E-15));
#10698=CARTESIAN_POINT('',(13.2909328553994,5.46084222270728,1.));
#10699=CARTESIAN_POINT('Origin',(8.4741241801467E-13,-0.080917771487827,
1.00000000000058));
#10700=CARTESIAN_POINT('',(13.2909328553994,5.46084222270728,4.11429224827654E-15));
#10701=CARTESIAN_POINT('Origin',(1.56125112837913E-14,-0.080917771488119,
1.));
#10702=CARTESIAN_POINT('',(-1.84616149105004,-14.362083261355,1.));
#10703=CARTESIAN_POINT('',(-1.16340283080869,-14.4338440882107,1.));
#10704=CARTESIAN_POINT('Origin',(-1.5710089479315E-13,-0.0809177714894745,
1.00000000000058));
#10705=CARTESIAN_POINT('',(-1.84616149105004,-14.362083261355,-0.999999999999996));
#10706=CARTESIAN_POINT('',(-1.84616149105004,-14.362083261355,4.11429224827654E-15));
#10707=CARTESIAN_POINT('',(-1.16340283080869,-14.4338440882107,-0.999999999999996));
#10708=CARTESIAN_POINT('Origin',(-1.5710089479315E-13,-0.0809177714894745,
-1.00000000000057));
#10709=CARTESIAN_POINT('',(-1.16340283080869,-14.4338440882107,4.11429224827654E-15));
#10710=CARTESIAN_POINT('Origin',(1.61979340522206E-14,-0.0809177714881199,
-0.999999999999996));
#10711=CARTESIAN_POINT('',(-9.03593732412197,-8.89675865936698,-0.999999999999996));
#10712=CARTESIAN_POINT('Origin',(-6.29005919429158,-11.3580426722998,-1.));
#10713=CARTESIAN_POINT('',(-9.03975952554573,-8.53215275344816,-0.999999999999996));
#10714=CARTESIAN_POINT('Origin',(-9.23699064246671,-8.71654333487274,-0.999999999999995));
#10715=CARTESIAN_POINT('',(-9.349850403976,-8.18776194312912,-0.999999999999996));
#10716=CARTESIAN_POINT('Origin',(-1.94202293135604E-12,-0.0809177714900912,
-0.999999999999996));
#10717=CARTESIAN_POINT('',(-9.71205943175173,-8.14584898508068,-0.999999999999996));
#10718=CARTESIAN_POINT('Origin',(-9.55384714006274,-8.36463854323765,-0.999999999999996));
#10719=CARTESIAN_POINT('Origin',(-11.8728378521018,-5.15773882741439,-0.999999999999996));
#10720=CARTESIAN_POINT('',(-10.6713967989502,-6.82543437723631,-0.999999999999996));
#10721=CARTESIAN_POINT('Origin',(-8.4972524150608,-9.80383359396352,-0.999999999999996));
#10722=CARTESIAN_POINT('',(-10.5993296457206,-6.46800130478777,-0.999999999999996));
#10723=CARTESIAN_POINT('Origin',(-10.8305877470818,-6.60735585460522,-0.999999999999996));
#10724=CARTESIAN_POINT('',(-10.8310414187911,-6.06666474111783,-0.999999999999996));
#10725=CARTESIAN_POINT('Origin',(1.26721549920106E-12,-0.0809177714874432,
-0.999999999999996));
#10726=CARTESIAN_POINT('',(-11.176621116299,-5.95036019036879,-0.999999999999996));
#10727=CARTESIAN_POINT('Origin',(-11.0673550497465,-6.19726285681884,-0.999999999999996));
#10728=CARTESIAN_POINT('Origin',(-12.6689183086518,-2.57829631406167,-1.));
#10729=CARTESIAN_POINT('',(-11.8404650266211,-4.45934235565306,-0.999999999999996));
#10730=CARTESIAN_POINT('Origin',(-10.3330749309508,-7.82468643845863,-0.999999999999996));
#10731=CARTESIAN_POINT('',(-11.6956581991509,-4.12470365709499,-0.999999999999996));
#10732=CARTESIAN_POINT('Origin',(-11.9508361962233,-4.21293171278095,-0.999999999999996));
#10733=CARTESIAN_POINT('',(-11.838863950502,-3.68396167373302,-0.999999999999996));
#10734=CARTESIAN_POINT('Origin',(9.35449634420493E-12,-0.0809177714850636,
-0.999999999999996));
#10735=CARTESIAN_POINT('',(-12.1527108266856,-3.49834859724226,-0.999999999999996));
#10736=CARTESIAN_POINT('Origin',(-12.0971664366948,-3.76257354069109,-0.999999999999996));
#10737=CARTESIAN_POINT('Origin',(-12.9113062428988,0.110293625353355,-1.));
#10738=CARTESIAN_POINT('',(-12.4920481157737,-1.90189216972961,-0.999999999999996));
#10739=CARTESIAN_POINT('Origin',(-11.7172924887636,-5.50709943348233,-0.999999999999996));
#10740=CARTESIAN_POINT('',(-12.2808303672837,-1.60467316196364,-0.999999999999996));
#10741=CARTESIAN_POINT('Origin',(-12.5487757571153,-1.63791873411946,-0.999999999999995));
#10742=CARTESIAN_POINT('',(-12.3292713184038,-1.14378829849724,-0.999999999999996));
#10743=CARTESIAN_POINT('Origin',(5.0558515707344E-12,-0.0809177714875954,
-0.999999999999996));
#10744=CARTESIAN_POINT('',(-12.5976687587696,-0.896978878377764,-0.999999999999996));
#10745=CARTESIAN_POINT('Origin',(-12.5982736017144,-1.16697820090472,-0.999999999999995));
#10746=CARTESIAN_POINT('Origin',(-12.5894081390099,2.79052670919229,-0.999999999999996));
#10747=CARTESIAN_POINT('',(-12.5976687587696,0.735143335401609,-0.999999999999996));
#10748=CARTESIAN_POINT('Origin',(-12.5894081390099,-2.95236225216844,-0.999999999999996));
#10749=CARTESIAN_POINT('',(-12.3292713184038,0.981952755521089,-0.999999999999996));
#10750=CARTESIAN_POINT('Origin',(-12.5982736017144,1.00514265792856,-0.999999999999996));
#10751=CARTESIAN_POINT('',(-12.2808303672836,1.44283761898748,-0.999999999999996));
#10752=CARTESIAN_POINT('Origin',(-2.37310171513627E-12,-0.0809177714879208,
-0.999999999999996));
#10753=CARTESIAN_POINT('',(-12.4920481157737,1.74005662675346,-0.999999999999996));
#10754=CARTESIAN_POINT('Origin',(-12.5487757571153,1.47608319114332,-0.999999999999996));
#10755=CARTESIAN_POINT('Origin',(-11.7172924887636,5.3452638905062,-1.));
#10756=CARTESIAN_POINT('',(-12.1527108266856,3.3365130542661,-0.999999999999996));
#10757=CARTESIAN_POINT('Origin',(-12.9113062428988,-0.272129168329482,-1.));
#10758=CARTESIAN_POINT('',(-11.838863950502,3.52212613075686,-0.999999999999996));
#10759=CARTESIAN_POINT('Origin',(-12.0971664366947,3.60073799771494,-0.999999999999996));
#10760=CARTESIAN_POINT('',(-11.6956581991509,3.96286811411883,-0.999999999999996));
#10761=CARTESIAN_POINT('Origin',(4.26828711264093E-12,-0.080917771489527,
-0.999999999999996));
#10762=CARTESIAN_POINT('',(-11.8404650266211,4.29750681267689,-0.999999999999996));
#10763=CARTESIAN_POINT('Origin',(-11.9508361962233,4.0510961698048,-0.999999999999996));
#10764=CARTESIAN_POINT('Origin',(-10.3330749309508,7.66285089548245,-0.999999999999996));
#10765=CARTESIAN_POINT('',(-11.176621116299,5.78852464739262,-0.999999999999996));
#10766=CARTESIAN_POINT('Origin',(-12.6689183086518,2.4164607710855,-1.));
#10767=CARTESIAN_POINT('',(-10.8310414187911,5.90482919814167,-0.999999999999996));
#10768=CARTESIAN_POINT('Origin',(-11.0673550497465,6.03542731384268,-0.999999999999996));
#10769=CARTESIAN_POINT('',(-10.5993296457206,6.30616576181161,-0.999999999999996));
#10770=CARTESIAN_POINT('Origin',(-1.49966844498195E-12,-0.0809177714873426,
-0.999999999999996));
#10771=CARTESIAN_POINT('',(-10.6713967989501,6.66359883426014,-0.999999999999996));
#10772=CARTESIAN_POINT('Origin',(-10.8305877470818,6.44552031162906,-0.999999999999996));
#10773=CARTESIAN_POINT('Origin',(-8.49725241506071,9.64199805098735,-0.999999999999996));
#10774=CARTESIAN_POINT('',(-9.71205943175167,7.98401344210451,-0.999999999999996));
#10775=CARTESIAN_POINT('Origin',(-11.8728378521018,4.99590328443823,-1.));
#10776=CARTESIAN_POINT('',(-9.34985040397594,8.02592640015294,-0.999999999999996));
#10777=CARTESIAN_POINT('Origin',(-9.55384714006268,8.20280300026148,-0.999999999999995));
#10778=CARTESIAN_POINT('',(-9.03975952554566,8.37031721047198,-0.999999999999996));
#10779=CARTESIAN_POINT('Origin',(-2.06258621293642E-12,-0.0809177714861846,
-0.999999999999996));
#10780=CARTESIAN_POINT('',(-9.03593732412191,8.7349231163908,-0.999999999999996));
#10781=CARTESIAN_POINT('Origin',(-9.23699064246666,8.55470779189656,-0.999999999999996));
#10782=CARTESIAN_POINT('Origin',(-6.29005919429155,11.1962071293236,-1.));
#10783=CARTESIAN_POINT('',(-7.82303414640506,9.82702604294875,-0.999999999999996));
#10784=CARTESIAN_POINT('Origin',(-10.557857409218,7.35346435635671,-0.999999999999996));
#10785=CARTESIAN_POINT('',(-7.46002606094707,9.79271561090918,-0.999999999999996));
#10786=CARTESIAN_POINT('Origin',(-7.62279026591319,10.0081403392524,-0.999999999999996));
#10787=CARTESIAN_POINT('',(-7.08510853652553,10.0651091368959,-0.999999999999996));
#10788=CARTESIAN_POINT('Origin',(4.36716635077161E-13,-0.080917771488739,
-0.999999999999996));
#10789=CARTESIAN_POINT('',(-7.00556402899164,10.4209528486231,-0.999999999999996));
#10790=CARTESIAN_POINT('Origin',(-7.239692722777,10.2864769967152,-0.999999999999996));
#10791=CARTESIAN_POINT('Origin',(-3.80796020367909,12.2575517358452,-0.999999999999996));
#10792=CARTESIAN_POINT('',(-5.5921047297778,11.2370139555128,-0.999999999999996));
#10793=CARTESIAN_POINT('Origin',(-8.78144793533072,9.38610725516491,-1.));
#10794=CARTESIAN_POINT('',(-5.24416278187814,11.1279796639051,-0.999999999999996));
#10795=CARTESIAN_POINT('Origin',(-5.3585808789373,11.3725374261318,-0.999999999999996));
#10796=CARTESIAN_POINT('',(-4.82080430633644,11.3164710013847,-0.999999999999996));
#10797=CARTESIAN_POINT('Origin',(-2.89265139619133E-13,-0.0809177714872558,
-0.999999999999996));
#10798=CARTESIAN_POINT('',(-4.66901396936854,11.6480004411903,-0.999999999999996));
#10799=CARTESIAN_POINT('Origin',(-4.92598549120196,11.5651413018838,-0.999999999999996));
#10800=CARTESIAN_POINT('Origin',(-1.15943507954541,12.7796460183509,-1.));
#10801=CARTESIAN_POINT('',(-3.11677350256359,12.1523539421449,-0.999999999999996));
#10802=CARTESIAN_POINT('Origin',(-6.62124704860712,11.0049957324822,-1.));
#10803=CARTESIAN_POINT('',(-2.79910442495618,11.9733611127169,-0.999999999999996));
#10804=CARTESIAN_POINT('Origin',(-2.86017579422795,12.2363635610995,-0.999999999999996));
#10805=CARTESIAN_POINT('',(-2.34580779517484,12.0697122857598,-0.999999999999996));
#10806=CARTESIAN_POINT('Origin',(-1.83013326715553E-13,-0.0809177714870919,
-0.999999999999996));
#10807=CARTESIAN_POINT('',(-2.12840559486928,12.3624380262694,-0.999999999999996));
#10808=CARTESIAN_POINT('Origin',(-2.39698905616047,12.3348169415543,-0.999999999999996));
#10809=CARTESIAN_POINT('Origin',(1.53976292115111,12.7396719514087,-0.999999999999996));
#10810=CARTESIAN_POINT('',(-0.505224317348839,12.5330412531408,-0.999999999999996));
#10811=CARTESIAN_POINT('Origin',(-4.17166589359098,12.1393765935609,-0.999999999999996));
#10812=CARTESIAN_POINT('',(-0.231711773070462,12.2919127314413,-0.999999999999996));
#10813=CARTESIAN_POINT('Origin',(-0.236767302664724,12.5618653969598,-0.999999999999996));
#10814=CARTESIAN_POINT('',(0.231711773070499,12.2919127314413,-0.999999999999996));
#10815=CARTESIAN_POINT('Origin',(1.82145964977565E-14,-0.0809177714804904,
-0.999999999999996));
#10816=CARTESIAN_POINT('',(0.505224317348871,12.5330412531408,-0.999999999999996));
#10817=CARTESIAN_POINT('Origin',(0.236767302664761,12.5618653969598,-0.999999999999996));
#10818=CARTESIAN_POINT('Origin',(4.17166589359101,12.1393765935609,-0.999999999999996));
#10819=CARTESIAN_POINT('',(2.79910442495637,11.9733611127168,-0.999999999999996));
#10820=CARTESIAN_POINT('Origin',(9.63855731339613E-13,-0.0809177714833623,
-0.999999999999996));
#10821=CARTESIAN_POINT('',(3.11677350256379,12.1523539421449,-0.999999999999996));
#10822=CARTESIAN_POINT('Origin',(2.86017579422815,12.2363635610995,-0.999999999999995));
#10823=CARTESIAN_POINT('Origin',(6.62124704860725,11.0049957324821,-0.999999999999996));
#10824=CARTESIAN_POINT('',(5.24416278187833,11.127979663905,-0.999999999999996));
#10825=CARTESIAN_POINT('Origin',(-9.87925019568792E-13,-0.0809177714904624,
-0.999999999999996));
#10826=CARTESIAN_POINT('',(5.59210472977799,11.2370139555127,-0.999999999999996));
#10827=CARTESIAN_POINT('Origin',(5.35858087893749,11.3725374261318,-0.999999999999996));
#10828=CARTESIAN_POINT('Origin',(8.78144793533089,9.38610725516478,-1.));
#10829=CARTESIAN_POINT('Origin',(3.80796020367927,12.2575517358452,-0.999999999999996));
#10830=CARTESIAN_POINT('',(7.46002606094724,9.79271561090908,-0.999999999999996));
#10831=CARTESIAN_POINT('Origin',(-7.51135265097957E-13,-0.0809177714892022,
-0.999999999999996));
#10832=CARTESIAN_POINT('',(7.82303414640522,9.82702604294864,-0.999999999999996));
#10833=CARTESIAN_POINT('Origin',(7.62279026591336,10.0081403392523,-0.999999999999996));
#10834=CARTESIAN_POINT('Origin',(10.5578574092182,7.35346435635655,-1.));
#10835=CARTESIAN_POINT('Origin',(6.29005919429175,11.1962071293235,-0.999999999999996));
#10836=CARTESIAN_POINT('',(9.34985040397608,8.02592640015281,-0.999999999999996));
#10837=CARTESIAN_POINT('Origin',(1.21430643318376E-14,-0.080917771488098,
-0.999999999999996));
#10838=CARTESIAN_POINT('',(9.71205943175181,7.98401344210438,-0.999999999999996));
#10839=CARTESIAN_POINT('Origin',(9.55384714006283,8.20280300026134,-0.999999999999995));
#10840=CARTESIAN_POINT('Origin',(11.8728378521019,4.99590328443808,-0.999999999999996));
#10841=CARTESIAN_POINT('Origin',(8.49725241506087,9.64199805098723,-1.));
#10842=CARTESIAN_POINT('',(10.8310414187912,5.90482919814151,-0.999999999999996));
#10843=CARTESIAN_POINT('Origin',(-4.47558656802016E-13,-0.0809177714884237,
-0.999999999999996));
#10844=CARTESIAN_POINT('',(11.1766211162991,5.78852464739247,-0.999999999999996));
#10845=CARTESIAN_POINT('Origin',(11.0673550497466,6.03542731384252,-0.999999999999996));
#10846=CARTESIAN_POINT('Origin',(12.6689183086518,2.41646077108533,-1.));
#10847=CARTESIAN_POINT('Origin',(10.3330749309509,7.66285089548231,-0.999999999999996));
#10848=CARTESIAN_POINT('',(11.838863950502,3.5221261307567,-0.999999999999996));
#10849=CARTESIAN_POINT('Origin',(1.47104550762833E-12,-0.0809177714876732,
-0.999999999999996));
#10850=CARTESIAN_POINT('',(12.1527108266857,3.33651305426593,-0.999999999999996));
#10851=CARTESIAN_POINT('Origin',(12.0971664366948,3.60073799771477,-0.999999999999996));
#10852=CARTESIAN_POINT('Origin',(12.9113062428988,-0.272129168329659,-0.999999999999996));
#10853=CARTESIAN_POINT('Origin',(11.7172924887637,5.345263890506,-1.));
#10854=CARTESIAN_POINT('',(12.3292713184039,0.981952755520918,-0.999999999999996));
#10855=CARTESIAN_POINT('Origin',(-1.40512601554121E-12,-0.0809177714882771,
-0.999999999999996));
#10856=CARTESIAN_POINT('',(12.5976687587696,0.735143335401439,-0.999999999999996));
#10857=CARTESIAN_POINT('Origin',(12.5982736017145,1.00514265792839,-0.999999999999996));
#10858=CARTESIAN_POINT('Origin',(12.5894081390099,-2.95236225216863,-1.));
#10859=CARTESIAN_POINT('',(12.5976687587696,-0.896978878377931,-0.999999999999996));
#10860=CARTESIAN_POINT('Origin',(12.58940813901,2.79052670919211,-0.999999999999996));
#10861=CARTESIAN_POINT('',(12.3292713184038,-1.14378829849741,-0.999999999999996));
#10862=CARTESIAN_POINT('Origin',(12.5982736017145,-1.16697820090489,-0.999999999999996));
#10863=CARTESIAN_POINT('Origin',(-5.25534477047174E-12,-0.08091777148747,
-0.999999999999996));
#10864=CARTESIAN_POINT('Origin',(11.7172924887636,-5.50709943348249,-0.999999999999996));
#10865=CARTESIAN_POINT('',(12.1527108266856,-3.49834859724242,-0.999999999999996));
#10866=CARTESIAN_POINT('Origin',(12.9113062428988,0.110293625353176,-1.));
#10867=CARTESIAN_POINT('',(11.838863950502,-3.68396167373318,-0.999999999999996));
#10868=CARTESIAN_POINT('Origin',(12.0971664366947,-3.76257354069125,-0.999999999999996));
#10869=CARTESIAN_POINT('Origin',(-2.20223145275256E-12,-0.0809177714873727,
-0.999999999999996));
#10870=CARTESIAN_POINT('Origin',(10.3330749309508,-7.82468643845877,-1.));
#10871=CARTESIAN_POINT('',(11.176621116299,-5.95036019036894,-0.999999999999996));
#10872=CARTESIAN_POINT('Origin',(12.6689183086518,-2.57829631406186,-0.999999999999996));
#10873=CARTESIAN_POINT('',(10.8310414187911,-6.06666474111799,-0.999999999999996));
#10874=CARTESIAN_POINT('Origin',(11.0673550497465,-6.197262856819,-0.999999999999996));
#10875=CARTESIAN_POINT('Origin',(2.35835656559047E-12,-0.0809177714894533,
-0.999999999999996));
#10876=CARTESIAN_POINT('Origin',(8.49725241506068,-9.80383359396365,-0.999999999999996));
#10877=CARTESIAN_POINT('',(9.71205943175165,-8.14584898508081,-0.999999999999996));
#10878=CARTESIAN_POINT('Origin',(11.8728378521018,-5.15773882741455,-1.));
#10879=CARTESIAN_POINT('',(9.34985040397592,-8.18776194312925,-0.999999999999996));
#10880=CARTESIAN_POINT('Origin',(9.55384714006266,-8.36463854323778,-0.999999999999996));
#10881=CARTESIAN_POINT('Origin',(1.0842021724855E-13,-0.0809177714881883,
-0.999999999999996));
#10882=CARTESIAN_POINT('Origin',(6.29005919429151,-11.3580426722999,-0.999999999999996));
#10883=CARTESIAN_POINT('',(7.82303414640502,-9.98886158592504,-0.999999999999996));
#10884=CARTESIAN_POINT('Origin',(10.557857409218,-7.51529989933299,-1.));
#10885=CARTESIAN_POINT('',(7.46002606094704,-9.95455115388547,-0.999999999999996));
#10886=CARTESIAN_POINT('Origin',(7.62279026591315,-10.1699758822287,-0.999999999999996));
#10887=CARTESIAN_POINT('Origin',(2.12937306676153E-13,-0.0809177714885291,
-0.999999999999996));
#10888=CARTESIAN_POINT('Origin',(3.80796020367903,-12.4193872788215,-0.999999999999996));
#10889=CARTESIAN_POINT('',(5.59210472977776,-11.3988494984891,-0.999999999999996));
#10890=CARTESIAN_POINT('Origin',(8.78144793533066,-9.54794279814123,-0.999999999999996));
#10891=CARTESIAN_POINT('',(5.2441627818781,-11.2898152068813,-0.999999999999996));
#10892=CARTESIAN_POINT('Origin',(5.35858087893726,-11.5343729691081,-0.999999999999996));
#10893=CARTESIAN_POINT('Origin',(-2.38004060904018E-12,-0.0809177714827325,
-0.999999999999996));
#10894=CARTESIAN_POINT('',(3.11677350256355,-12.3141894851212,-0.999999999999996));
#10895=CARTESIAN_POINT('Origin',(6.62124704860706,-11.1668312754584,-1.));
#10896=CARTESIAN_POINT('',(2.79910442495613,-12.1351966556931,-0.999999999999996));
#10897=CARTESIAN_POINT('Origin',(2.8601757942279,-12.3981991040758,-0.999999999999996));
#10898=CARTESIAN_POINT('Origin',(-5.72241906637849E-13,-0.0809177714854283,
-0.999999999999996));
#10899=CARTESIAN_POINT('',(1.16340283080872,-14.4338440882107,-0.999999999999996));
#10900=CARTESIAN_POINT('Origin',(9.19403442267708E-14,-0.0809177714883105,
-1.00000000000057));
#10901=CARTESIAN_POINT('',(0.505224317348871,-12.694876796117,-0.999999999999996));
#10902=CARTESIAN_POINT('Origin',(4.17166589359103,-12.3012121365371,-1.));
#10903=CARTESIAN_POINT('',(0.231711773070495,-12.4537482744175,-0.999999999999996));
#10904=CARTESIAN_POINT('Origin',(0.23676730266476,-12.723700939936,-0.999999999999996));
#10905=CARTESIAN_POINT('',(-0.231711773070466,-12.4537482744175,-0.999999999999996));
#10906=CARTESIAN_POINT('Origin',(1.27664805810168E-14,-0.0809177714956016,
-0.999999999999996));
#10907=CARTESIAN_POINT('',(-0.505224317348839,-12.694876796117,-0.999999999999996));
#10908=CARTESIAN_POINT('Origin',(-0.236767302664738,-12.723700939936,-0.999999999999996));
#10909=CARTESIAN_POINT('Origin',(-4.171665893591,-12.3012121365371,-0.999999999999996));
#10910=CARTESIAN_POINT('',(-2.12840559486936,-12.5242735692457,-0.999999999999996));
#10911=CARTESIAN_POINT('Origin',(1.53976292115102,-12.9015074943849,-0.999999999999996));
#10912=CARTESIAN_POINT('',(-2.34580779517493,-12.231547828736,-0.999999999999996));
#10913=CARTESIAN_POINT('Origin',(-2.39698905616056,-12.4966524845305,-0.999999999999996));
#10914=CARTESIAN_POINT('',(-2.79910442495626,-12.1351966556931,-0.999999999999996));
#10915=CARTESIAN_POINT('Origin',(6.0281640790194E-13,-0.0809177714853745,
-0.999999999999996));
#10916=CARTESIAN_POINT('',(-3.11677350256368,-12.3141894851212,-0.999999999999996));
#10917=CARTESIAN_POINT('Origin',(-2.86017579422803,-12.3981991040758,-0.999999999999996));
#10918=CARTESIAN_POINT('Origin',(-6.62124704860716,-11.1668312754584,-0.999999999999996));
#10919=CARTESIAN_POINT('',(-4.66901396936862,-11.8098359841665,-0.999999999999996));
#10920=CARTESIAN_POINT('Origin',(-1.15943507954551,-12.9414815613271,-1.));
#10921=CARTESIAN_POINT('',(-4.82080430633652,-11.4783065443609,-0.999999999999996));
#10922=CARTESIAN_POINT('Origin',(-4.92598549120204,-11.72697684486,-0.999999999999996));
#10923=CARTESIAN_POINT('',(-5.24416278187822,-11.2898152068813,-0.999999999999996));
#10924=CARTESIAN_POINT('Origin',(2.17707796235089E-13,-0.0809177714876878,
-0.999999999999996));
#10925=CARTESIAN_POINT('',(-5.59210472977788,-11.398849498489,-0.999999999999996));
#10926=CARTESIAN_POINT('Origin',(-5.35858087893738,-11.534372969108,-0.999999999999996));
#10927=CARTESIAN_POINT('Origin',(-8.78144793533077,-9.54794279814109,-0.999999999999996));
#10928=CARTESIAN_POINT('',(-7.00556402899171,-10.5827883915993,-0.999999999999996));
#10929=CARTESIAN_POINT('Origin',(-3.80796020367914,-12.4193872788215,-1.));
#10930=CARTESIAN_POINT('',(-7.0851085365256,-10.2269446798721,-0.999999999999996));
#10931=CARTESIAN_POINT('Origin',(-7.23969272277707,-10.4483125396914,-0.999999999999996));
#10932=CARTESIAN_POINT('',(-7.46002606094714,-9.95455115388536,-0.999999999999996));
#10933=CARTESIAN_POINT('Origin',(-1.9298798670242E-13,-0.0809177714885872,
-0.999999999999996));
#10934=CARTESIAN_POINT('',(-7.82303414640512,-9.98886158592494,-0.999999999999996));
#10935=CARTESIAN_POINT('Origin',(-7.62279026591326,-10.1699758822286,-0.999999999999996));
#10936=CARTESIAN_POINT('Origin',(-10.5578574092181,-7.51529989933288,-0.999999999999996));
#10937=CARTESIAN_POINT('',(-0.749999999999984,3.66908222851188,-0.999999999999996));
#10938=CARTESIAN_POINT('',(-0.749999999999984,3.66908222851188,-0.999999999999996));
#10939=CARTESIAN_POINT('',(0.750000000000016,3.66908222851188,-0.999999999999996));
#10940=CARTESIAN_POINT('',(0.750000000000016,3.66908222851188,-0.999999999999996));
#10941=CARTESIAN_POINT('',(-0.749999999999984,3.66908222851188,-0.999999999999996));
#10942=CARTESIAN_POINT('Origin',(1.61979340522206E-14,-0.0809177714881199,
1.));
#10943=CARTESIAN_POINT('',(-9.03593732412197,-8.89675865936698,1.));
#10944=CARTESIAN_POINT('Origin',(-6.29005919429161,-11.3580426722998,1.));
#10945=CARTESIAN_POINT('',(-7.82303414640512,-9.98886158592494,1.));
#10946=CARTESIAN_POINT('Origin',(-10.5578574092181,-7.51529989933286,1.00000000000001));
#10947=CARTESIAN_POINT('',(-7.46002606094714,-9.95455115388536,1.));
#10948=CARTESIAN_POINT('Origin',(-7.62279026591326,-10.1699758822286,1.));
#10949=CARTESIAN_POINT('',(-7.0851085365256,-10.2269446798721,1.));
#10950=CARTESIAN_POINT('Origin',(-1.9298798670242E-13,-0.0809177714885872,
1.));
#10951=CARTESIAN_POINT('',(-7.00556402899171,-10.5827883915993,1.));
#10952=CARTESIAN_POINT('Origin',(-7.23969272277707,-10.4483125396914,1.));
#10953=CARTESIAN_POINT('Origin',(-3.80796020367915,-12.4193872788215,1.));
#10954=CARTESIAN_POINT('',(-5.59210472977788,-11.398849498489,1.));
#10955=CARTESIAN_POINT('Origin',(-8.78144793533078,-9.54794279814109,1.));
#10956=CARTESIAN_POINT('',(-5.24416278187822,-11.2898152068813,1.));
#10957=CARTESIAN_POINT('Origin',(-5.35858087893738,-11.534372969108,1.));
#10958=CARTESIAN_POINT('',(-4.82080430633652,-11.4783065443609,1.));
#10959=CARTESIAN_POINT('Origin',(2.17707796235089E-13,-0.0809177714876878,
1.));
#10960=CARTESIAN_POINT('',(-4.66901396936862,-11.8098359841665,1.));
#10961=CARTESIAN_POINT('Origin',(-4.92598549120204,-11.72697684486,1.));
#10962=CARTESIAN_POINT('Origin',(-1.15943507954552,-12.9414815613271,1.00000000000001));
#10963=CARTESIAN_POINT('',(-3.11677350256368,-12.3141894851212,1.));
#10964=CARTESIAN_POINT('Origin',(-6.62124704860717,-11.1668312754584,1.00000000000001));
#10965=CARTESIAN_POINT('',(-2.79910442495626,-12.1351966556931,1.));
#10966=CARTESIAN_POINT('Origin',(-2.86017579422803,-12.3981991040758,1.));
#10967=CARTESIAN_POINT('',(-2.34580779517493,-12.231547828736,1.));
#10968=CARTESIAN_POINT('Origin',(6.0281640790194E-13,-0.0809177714853745,
1.));
#10969=CARTESIAN_POINT('',(-2.12840559486936,-12.5242735692457,1.));
#10970=CARTESIAN_POINT('Origin',(-2.39698905616056,-12.4966524845305,1.));
#10971=CARTESIAN_POINT('Origin',(1.53976292115103,-12.9015074943849,1.00000000000001));
#10972=CARTESIAN_POINT('',(-0.505224317348839,-12.694876796117,1.));
#10973=CARTESIAN_POINT('Origin',(-4.171665893591,-12.3012121365371,1.));
#10974=CARTESIAN_POINT('',(-0.231711773070466,-12.4537482744175,1.));
#10975=CARTESIAN_POINT('Origin',(-0.236767302664738,-12.723700939936,1.));
#10976=CARTESIAN_POINT('',(0.231711773070495,-12.4537482744175,1.));
#10977=CARTESIAN_POINT('Origin',(1.27664805810168E-14,-0.0809177714956016,
1.));
#10978=CARTESIAN_POINT('',(0.505224317348871,-12.694876796117,1.));
#10979=CARTESIAN_POINT('Origin',(0.23676730266476,-12.723700939936,1.));
#10980=CARTESIAN_POINT('',(1.16340283080871,-14.4338440882107,1.));
#10981=CARTESIAN_POINT('Origin',(4.17166589359103,-12.3012121365371,1.));
#10982=CARTESIAN_POINT('Origin',(4.2858511878352E-13,-0.0809177714923429,
1.00000000000058));
#10983=CARTESIAN_POINT('',(2.79910442495613,-12.1351966556931,1.));
#10984=CARTESIAN_POINT('Origin',(-5.72241906637849E-13,-0.0809177714854283,
1.));
#10985=CARTESIAN_POINT('',(3.11677350256355,-12.3141894851212,1.));
#10986=CARTESIAN_POINT('Origin',(2.8601757942279,-12.3981991040758,1.));
#10987=CARTESIAN_POINT('Origin',(6.62124704860705,-11.1668312754585,1.));
#10988=CARTESIAN_POINT('',(5.2441627818781,-11.2898152068813,1.));
#10989=CARTESIAN_POINT('Origin',(-2.38004060904018E-12,-0.0809177714827325,
1.));
#10990=CARTESIAN_POINT('',(5.59210472977776,-11.3988494984891,1.));
#10991=CARTESIAN_POINT('Origin',(5.35858087893726,-11.5343729691081,1.));
#10992=CARTESIAN_POINT('Origin',(8.78144793533065,-9.54794279814124,1.));
#10993=CARTESIAN_POINT('Origin',(3.80796020367901,-12.4193872788215,1.));
#10994=CARTESIAN_POINT('',(7.46002606094704,-9.95455115388547,1.));
#10995=CARTESIAN_POINT('Origin',(2.12937306676153E-13,-0.0809177714885291,
1.));
#10996=CARTESIAN_POINT('',(7.82303414640502,-9.98886158592504,1.));
#10997=CARTESIAN_POINT('Origin',(7.62279026591315,-10.1699758822287,1.));
#10998=CARTESIAN_POINT('Origin',(10.557857409218,-7.515299899333,1.00000000000001));
#10999=CARTESIAN_POINT('Origin',(6.29005919429151,-11.3580426722999,1.));
#11000=CARTESIAN_POINT('',(9.34985040397592,-8.18776194312925,1.));
#11001=CARTESIAN_POINT('Origin',(1.0842021724855E-13,-0.0809177714881883,
1.));
#11002=CARTESIAN_POINT('',(9.71205943175165,-8.14584898508081,1.));
#11003=CARTESIAN_POINT('Origin',(9.55384714006266,-8.36463854323778,1.));
#11004=CARTESIAN_POINT('Origin',(11.8728378521018,-5.15773882741455,1.));
#11005=CARTESIAN_POINT('Origin',(8.49725241506067,-9.80383359396364,1.));
#11006=CARTESIAN_POINT('',(10.8310414187911,-6.06666474111799,1.));
#11007=CARTESIAN_POINT('Origin',(2.35835656559047E-12,-0.0809177714894533,
1.));
#11008=CARTESIAN_POINT('',(11.176621116299,-5.95036019036894,1.));
#11009=CARTESIAN_POINT('Origin',(11.0673550497465,-6.197262856819,1.));
#11010=CARTESIAN_POINT('Origin',(12.6689183086518,-2.57829631406185,1.));
#11011=CARTESIAN_POINT('Origin',(10.3330749309508,-7.82468643845875,1.));
#11012=CARTESIAN_POINT('',(11.838863950502,-3.68396167373318,1.));
#11013=CARTESIAN_POINT('Origin',(-2.20223145275256E-12,-0.0809177714873727,
1.));
#11014=CARTESIAN_POINT('',(12.1527108266856,-3.49834859724242,1.));
#11015=CARTESIAN_POINT('Origin',(12.0971664366947,-3.76257354069125,1.));
#11016=CARTESIAN_POINT('Origin',(12.9113062428988,0.11029362535318,1.00000000000001));
#11017=CARTESIAN_POINT('Origin',(11.7172924887636,-5.50709943348251,1.00000000000001));
#11018=CARTESIAN_POINT('',(12.3292713184038,-1.14378829849741,1.));
#11019=CARTESIAN_POINT('Origin',(-5.25534477047174E-12,-0.08091777148747,
1.));
#11020=CARTESIAN_POINT('',(12.5976687587696,-0.896978878377931,1.));
#11021=CARTESIAN_POINT('Origin',(12.5982736017145,-1.16697820090489,1.));
#11022=CARTESIAN_POINT('Origin',(12.58940813901,2.79052670919212,1.));
#11023=CARTESIAN_POINT('',(12.5976687587696,0.735143335401439,1.));
#11024=CARTESIAN_POINT('Origin',(12.5894081390099,-2.95236225216863,1.00000000000001));
#11025=CARTESIAN_POINT('',(12.3292713184039,0.981952755520918,1.));
#11026=CARTESIAN_POINT('Origin',(12.5982736017145,1.00514265792839,1.));
#11027=CARTESIAN_POINT('Origin',(-1.40512601554121E-12,-0.0809177714882771,
1.));
#11028=CARTESIAN_POINT('Origin',(11.7172924887637,5.345263890506,1.));
#11029=CARTESIAN_POINT('',(12.1527108266857,3.33651305426593,1.));
#11030=CARTESIAN_POINT('Origin',(12.9113062428988,-0.272129168329664,1.00000000000001));
#11031=CARTESIAN_POINT('',(11.838863950502,3.5221261307567,1.));
#11032=CARTESIAN_POINT('Origin',(12.0971664366948,3.60073799771477,1.));
#11033=CARTESIAN_POINT('Origin',(1.47104550762833E-12,-0.0809177714876732,
1.));
#11034=CARTESIAN_POINT('Origin',(10.3330749309509,7.66285089548231,1.));
#11035=CARTESIAN_POINT('',(11.1766211162991,5.78852464739247,1.));
#11036=CARTESIAN_POINT('Origin',(12.6689183086518,2.41646077108532,1.00000000000001));
#11037=CARTESIAN_POINT('',(10.8310414187912,5.90482919814151,1.));
#11038=CARTESIAN_POINT('Origin',(11.0673550497466,6.03542731384252,1.));
#11039=CARTESIAN_POINT('Origin',(-4.47558656802016E-13,-0.0809177714884237,
1.));
#11040=CARTESIAN_POINT('Origin',(8.49725241506088,9.64199805098721,1.));
#11041=CARTESIAN_POINT('',(9.71205943175181,7.98401344210438,1.));
#11042=CARTESIAN_POINT('Origin',(11.8728378521019,4.99590328443805,1.00000000000001));
#11043=CARTESIAN_POINT('',(9.34985040397608,8.02592640015281,1.));
#11044=CARTESIAN_POINT('Origin',(9.55384714006283,8.20280300026134,1.));
#11045=CARTESIAN_POINT('Origin',(1.21430643318376E-14,-0.080917771488098,
1.));
#11046=CARTESIAN_POINT('Origin',(6.29005919429173,11.1962071293235,1.00000000000001));
#11047=CARTESIAN_POINT('',(7.82303414640522,9.82702604294864,1.));
#11048=CARTESIAN_POINT('Origin',(10.5578574092182,7.35346435635655,1.00000000000001));
#11049=CARTESIAN_POINT('',(7.46002606094724,9.79271561090908,1.));
#11050=CARTESIAN_POINT('Origin',(7.62279026591336,10.0081403392523,1.));
#11051=CARTESIAN_POINT('Origin',(-7.51135265097957E-13,-0.0809177714892022,
1.));
#11052=CARTESIAN_POINT('Origin',(3.80796020367927,12.2575517358452,1.));
#11053=CARTESIAN_POINT('',(5.59210472977799,11.2370139555127,1.));
#11054=CARTESIAN_POINT('Origin',(8.78144793533088,9.38610725516479,1.));
#11055=CARTESIAN_POINT('',(5.24416278187833,11.127979663905,1.));
#11056=CARTESIAN_POINT('Origin',(5.35858087893749,11.3725374261318,1.));
#11057=CARTESIAN_POINT('Origin',(-9.87925019568792E-13,-0.0809177714904624,
1.));
#11058=CARTESIAN_POINT('',(3.11677350256379,12.1523539421449,1.));
#11059=CARTESIAN_POINT('Origin',(6.62124704860725,11.0049957324821,1.));
#11060=CARTESIAN_POINT('',(2.79910442495637,11.9733611127168,1.));
#11061=CARTESIAN_POINT('Origin',(2.86017579422815,12.2363635610995,1.));
#11062=CARTESIAN_POINT('Origin',(9.63855731339613E-13,-0.0809177714833623,
1.));
#11063=CARTESIAN_POINT('',(0.505224317348871,12.5330412531408,1.));
#11064=CARTESIAN_POINT('Origin',(4.17166589359102,12.1393765935609,1.00000000000001));
#11065=CARTESIAN_POINT('',(0.231711773070499,12.2919127314413,1.));
#11066=CARTESIAN_POINT('Origin',(0.236767302664761,12.5618653969598,1.));
#11067=CARTESIAN_POINT('',(-0.231711773070462,12.2919127314413,1.));
#11068=CARTESIAN_POINT('Origin',(1.82145964977565E-14,-0.0809177714804904,
1.));
#11069=CARTESIAN_POINT('',(-0.505224317348839,12.5330412531408,1.));
#11070=CARTESIAN_POINT('Origin',(-0.236767302664724,12.5618653969598,1.));
#11071=CARTESIAN_POINT('Origin',(-4.17166589359098,12.1393765935609,1.));
#11072=CARTESIAN_POINT('',(-2.12840559486928,12.3624380262694,1.));
#11073=CARTESIAN_POINT('Origin',(1.53976292115111,12.7396719514087,1.));
#11074=CARTESIAN_POINT('',(-2.34580779517484,12.0697122857598,1.));
#11075=CARTESIAN_POINT('Origin',(-2.39698905616047,12.3348169415543,1.));
#11076=CARTESIAN_POINT('',(-2.79910442495618,11.9733611127169,1.));
#11077=CARTESIAN_POINT('Origin',(-1.83013326715553E-13,-0.0809177714870919,
1.));
#11078=CARTESIAN_POINT('',(-3.11677350256359,12.1523539421449,1.));
#11079=CARTESIAN_POINT('Origin',(-2.86017579422795,12.2363635610995,1.));
#11080=CARTESIAN_POINT('Origin',(-6.62124704860709,11.0049957324822,1.));
#11081=CARTESIAN_POINT('',(-4.66901396936854,11.6480004411903,1.));
#11082=CARTESIAN_POINT('Origin',(-1.15943507954541,12.7796460183509,1.00000000000001));
#11083=CARTESIAN_POINT('',(-4.82080430633644,11.3164710013847,1.));
#11084=CARTESIAN_POINT('Origin',(-4.92598549120196,11.5651413018838,1.));
#11085=CARTESIAN_POINT('',(-5.24416278187814,11.1279796639051,1.));
#11086=CARTESIAN_POINT('Origin',(-2.89265139619133E-13,-0.0809177714872558,
1.));
#11087=CARTESIAN_POINT('',(-5.5921047297778,11.2370139555128,1.));
#11088=CARTESIAN_POINT('Origin',(-5.3585808789373,11.3725374261318,1.));
#11089=CARTESIAN_POINT('Origin',(-8.78144793533071,9.38610725516491,1.));
#11090=CARTESIAN_POINT('',(-7.00556402899164,10.4209528486231,1.));
#11091=CARTESIAN_POINT('Origin',(-3.80796020367908,12.2575517358452,1.00000000000001));
#11092=CARTESIAN_POINT('',(-7.08510853652553,10.0651091368959,1.));
#11093=CARTESIAN_POINT('Origin',(-7.239692722777,10.2864769967152,1.));
#11094=CARTESIAN_POINT('',(-7.46002606094707,9.79271561090918,1.));
#11095=CARTESIAN_POINT('Origin',(4.36716635077161E-13,-0.080917771488739,
1.));
#11096=CARTESIAN_POINT('',(-7.82303414640506,9.82702604294875,1.));
#11097=CARTESIAN_POINT('Origin',(-7.62279026591319,10.0081403392524,1.));
#11098=CARTESIAN_POINT('Origin',(-10.557857409218,7.3534643563567,1.));
#11099=CARTESIAN_POINT('',(-9.03593732412191,8.7349231163908,1.));
#11100=CARTESIAN_POINT('Origin',(-6.29005919429155,11.1962071293236,1.00000000000001));
#11101=CARTESIAN_POINT('',(-9.03975952554566,8.37031721047198,1.));
#11102=CARTESIAN_POINT('Origin',(-9.23699064246666,8.55470779189656,1.));
#11103=CARTESIAN_POINT('',(-9.34985040397594,8.02592640015294,1.));
#11104=CARTESIAN_POINT('Origin',(-2.06258621293642E-12,-0.0809177714861846,
1.));
#11105=CARTESIAN_POINT('',(-9.71205943175167,7.98401344210451,1.));
#11106=CARTESIAN_POINT('Origin',(-9.55384714006268,8.20280300026148,1.));
#11107=CARTESIAN_POINT('Origin',(-11.8728378521018,4.99590328443823,1.));
#11108=CARTESIAN_POINT('',(-10.6713967989501,6.66359883426014,1.));
#11109=CARTESIAN_POINT('Origin',(-8.49725241506071,9.64199805098735,1.));
#11110=CARTESIAN_POINT('',(-10.5993296457206,6.30616576181161,1.));
#11111=CARTESIAN_POINT('Origin',(-10.8305877470818,6.44552031162906,1.));
#11112=CARTESIAN_POINT('',(-10.8310414187911,5.90482919814167,1.));
#11113=CARTESIAN_POINT('Origin',(-1.49966844498195E-12,-0.0809177714873426,
1.));
#11114=CARTESIAN_POINT('',(-11.176621116299,5.78852464739262,1.));
#11115=CARTESIAN_POINT('Origin',(-11.0673550497465,6.03542731384268,1.));
#11116=CARTESIAN_POINT('Origin',(-12.6689183086518,2.41646077108552,1.));
#11117=CARTESIAN_POINT('',(-11.8404650266211,4.29750681267689,1.));
#11118=CARTESIAN_POINT('Origin',(-10.3330749309508,7.66285089548245,1.));
#11119=CARTESIAN_POINT('',(-11.6956581991509,3.96286811411883,1.));
#11120=CARTESIAN_POINT('Origin',(-11.9508361962233,4.0510961698048,1.));
#11121=CARTESIAN_POINT('',(-11.838863950502,3.52212613075686,1.));
#11122=CARTESIAN_POINT('Origin',(4.26828711264093E-12,-0.080917771489527,
1.));
#11123=CARTESIAN_POINT('',(-12.1527108266856,3.3365130542661,1.));
#11124=CARTESIAN_POINT('Origin',(-12.0971664366947,3.60073799771494,1.));
#11125=CARTESIAN_POINT('Origin',(-12.9113062428988,-0.272129168329465,1.));
#11126=CARTESIAN_POINT('',(-12.4920481157737,1.74005662675346,1.));
#11127=CARTESIAN_POINT('Origin',(-11.7172924887636,5.3452638905062,1.00000000000001));
#11128=CARTESIAN_POINT('',(-12.2808303672836,1.44283761898748,1.));
#11129=CARTESIAN_POINT('Origin',(-12.5487757571153,1.47608319114332,1.));
#11130=CARTESIAN_POINT('',(-12.3292713184038,0.981952755521089,1.));
#11131=CARTESIAN_POINT('Origin',(-2.37310171513627E-12,-0.0809177714879208,
1.));
#11132=CARTESIAN_POINT('',(-12.5976687587696,0.735143335401609,1.));
#11133=CARTESIAN_POINT('Origin',(-12.5982736017144,1.00514265792856,1.));
#11134=CARTESIAN_POINT('Origin',(-12.5894081390099,-2.95236225216843,1.));
#11135=CARTESIAN_POINT('',(-12.5976687587696,-0.896978878377764,1.));
#11136=CARTESIAN_POINT('Origin',(-12.5894081390099,2.79052670919229,1.));
#11137=CARTESIAN_POINT('',(-12.3292713184038,-1.14378829849724,1.));
#11138=CARTESIAN_POINT('Origin',(-12.5982736017144,-1.16697820090472,1.));
#11139=CARTESIAN_POINT('',(-12.2808303672837,-1.60467316196364,1.));
#11140=CARTESIAN_POINT('Origin',(5.0558515707344E-12,-0.0809177714875954,
1.));
#11141=CARTESIAN_POINT('',(-12.4920481157737,-1.90189216972961,1.));
#11142=CARTESIAN_POINT('Origin',(-12.5487757571153,-1.63791873411946,1.));
#11143=CARTESIAN_POINT('Origin',(-11.7172924887636,-5.50709943348232,1.));
#11144=CARTESIAN_POINT('',(-12.1527108266856,-3.49834859724226,1.));
#11145=CARTESIAN_POINT('Origin',(-12.9113062428988,0.110293625353339,1.00000000000001));
#11146=CARTESIAN_POINT('',(-11.838863950502,-3.68396167373302,1.));
#11147=CARTESIAN_POINT('Origin',(-12.0971664366948,-3.76257354069109,1.));
#11148=CARTESIAN_POINT('',(-11.6956581991509,-4.12470365709499,1.));
#11149=CARTESIAN_POINT('Origin',(9.35449634420493E-12,-0.0809177714850636,
1.));
#11150=CARTESIAN_POINT('',(-11.8404650266211,-4.45934235565306,1.));
#11151=CARTESIAN_POINT('Origin',(-11.9508361962233,-4.21293171278095,1.));
#11152=CARTESIAN_POINT('Origin',(-10.3330749309508,-7.82468643845864,1.));
#11153=CARTESIAN_POINT('',(-11.176621116299,-5.95036019036879,1.));
#11154=CARTESIAN_POINT('Origin',(-12.6689183086518,-2.57829631406167,1.00000000000001));
#11155=CARTESIAN_POINT('',(-10.8310414187911,-6.06666474111783,1.));
#11156=CARTESIAN_POINT('Origin',(-11.0673550497465,-6.19726285681884,1.));
#11157=CARTESIAN_POINT('',(-10.5993296457206,-6.46800130478777,1.));
#11158=CARTESIAN_POINT('Origin',(1.26721549920106E-12,-0.0809177714874432,
1.));
#11159=CARTESIAN_POINT('',(-10.6713967989502,-6.82543437723631,1.));
#11160=CARTESIAN_POINT('Origin',(-10.8305877470818,-6.60735585460522,1.));
#11161=CARTESIAN_POINT('Origin',(-8.49725241506079,-9.80383359396352,1.));
#11162=CARTESIAN_POINT('',(-9.71205943175173,-8.14584898508068,1.));
#11163=CARTESIAN_POINT('Origin',(-11.8728378521018,-5.15773882741439,1.));
#11164=CARTESIAN_POINT('',(-9.349850403976,-8.18776194312912,1.));
#11165=CARTESIAN_POINT('Origin',(-9.55384714006274,-8.36463854323765,1.));
#11166=CARTESIAN_POINT('',(-9.03975952554573,-8.53215275344816,1.));
#11167=CARTESIAN_POINT('Origin',(-1.94202293135604E-12,-0.0809177714900912,
1.));
#11168=CARTESIAN_POINT('Origin',(-9.23699064246671,-8.71654333487274,1.));
#11169=CARTESIAN_POINT('',(-0.749999999999984,3.66908222851188,1.));
#11170=CARTESIAN_POINT('',(-0.749999999999984,3.66908222851188,1.));
#11171=CARTESIAN_POINT('',(0.750000000000016,3.66908222851188,1.));
#11172=CARTESIAN_POINT('',(-0.749999999999984,3.66908222851188,1.));
#11173=CARTESIAN_POINT('',(0.750000000000016,3.66908222851188,1.));
#11174=CARTESIAN_POINT('Origin',(1.56125112837913E-14,-0.080917771488119,
1.));
#11175=CARTESIAN_POINT('',(1.16340283080872,-14.4338440882107,4.11429224827654E-15));
#11176=CARTESIAN_POINT('Origin',(-4.17166589359099,-12.3012121365371,-0.999999999999996));
#11177=CARTESIAN_POINT('',(-0.505224317348839,-12.694876796117,-0.999999999999996));
#11178=CARTESIAN_POINT('Origin',(4.17166589359102,-12.3012121365371,-0.999999999999996));
#11179=CARTESIAN_POINT('',(0.50522431734887,-12.694876796117,-0.999999999999996));
#11180=CARTESIAN_POINT('Origin',(1.56125112837913E-14,-0.0809177714881191,
-0.999999999999996));
#11181=CARTESIAN_POINT('',(-0.231711773070466,-12.4537482744175,-0.999999999999996));
#11182=CARTESIAN_POINT('',(0.231711773070495,-12.4537482744175,-0.999999999999996));
#11183=CARTESIAN_POINT('Origin',(-0.236767302664731,-12.723700939936,-0.999999999999996));
#11184=CARTESIAN_POINT('Origin',(0.23676730266476,-12.723700939936,-0.999999999999996));
#11185=CARTESIAN_POINT('Origin',(1.53976292115102,-12.9015074943849,-0.999999999999996));
#11186=CARTESIAN_POINT('',(-2.12840559486936,-12.5242735692457,-0.999999999999996));
#11187=CARTESIAN_POINT('Origin',(-6.62124704860716,-11.1668312754584,-0.999999999999996));
#11188=CARTESIAN_POINT('',(-3.11677350256368,-12.3141894851212,-0.999999999999996));
#11189=CARTESIAN_POINT('Origin',(-2.86017579422803,-12.3981991040758,-0.999999999999996));
#11190=CARTESIAN_POINT('',(-2.79910442495626,-12.1351966556931,-0.999999999999996));
#11191=CARTESIAN_POINT('Origin',(1.56125112837913E-14,-0.0809177714881191,
-0.999999999999996));
#11192=CARTESIAN_POINT('',(-2.34580779517493,-12.231547828736,-0.999999999999996));
#11193=CARTESIAN_POINT('Origin',(-2.39698905616056,-12.4966524845305,-0.999999999999996));
#11194=CARTESIAN_POINT('Origin',(10.3330749309509,7.66285089548231,-0.999999999999996));
#11195=CARTESIAN_POINT('Origin',(12.9113062428988,-0.272129168329664,-0.999999999999996));
#11196=CARTESIAN_POINT('',(12.1527108266857,3.33651305426593,-0.999999999999996));
#11197=CARTESIAN_POINT('Origin',(12.0971664366948,3.60073799771476,-0.999999999999996));
#11198=CARTESIAN_POINT('',(11.838863950502,3.5221261307567,-0.999999999999996));
#11199=CARTESIAN_POINT('Origin',(1.56125112837913E-14,-0.0809177714881191,
-0.999999999999996));
#11200=CARTESIAN_POINT('Origin',(8.49725241506087,9.64199805098723,-0.999999999999996));
#11201=CARTESIAN_POINT('Origin',(12.6689183086518,2.41646077108535,-0.999999999999996));
#11202=CARTESIAN_POINT('',(11.1766211162991,5.78852464739247,-0.999999999999996));
#11203=CARTESIAN_POINT('Origin',(11.0673550497466,6.03542731384252,-0.999999999999996));
#11204=CARTESIAN_POINT('',(10.8310414187912,5.90482919814151,-0.999999999999996));
#11205=CARTESIAN_POINT('Origin',(1.56125112837913E-14,-0.0809177714881191,
-0.999999999999996));
#11206=CARTESIAN_POINT('Origin',(3.80796020367927,12.2575517358452,-0.999999999999996));
#11207=CARTESIAN_POINT('Origin',(10.5578574092182,7.35346435635656,-0.999999999999996));
#11208=CARTESIAN_POINT('',(7.82303414640522,9.82702604294864,-0.999999999999996));
#11209=CARTESIAN_POINT('Origin',(7.62279026591336,10.0081403392523,-0.999999999999996));
#11210=CARTESIAN_POINT('',(7.46002606094724,9.79271561090908,-0.999999999999996));
#11211=CARTESIAN_POINT('Origin',(1.56125112837913E-14,-0.0809177714881191,
-0.999999999999996));
#11212=CARTESIAN_POINT('Origin',(6.29005919429173,11.1962071293235,-0.999999999999996));
#11213=CARTESIAN_POINT('Origin',(11.8728378521019,4.99590328443808,-0.999999999999996));
#11214=CARTESIAN_POINT('',(9.71205943175181,7.98401344210438,-0.999999999999996));
#11215=CARTESIAN_POINT('Origin',(9.55384714006284,8.20280300026134,-0.999999999999996));
#11216=CARTESIAN_POINT('',(9.34985040397608,8.02592640015281,-0.999999999999996));
#11217=CARTESIAN_POINT('Origin',(1.56125112837913E-14,-0.0809177714881191,
-0.999999999999996));
#11218=CARTESIAN_POINT('Origin',(11.7172924887637,5.34526389050601,-0.999999999999996));
#11219=CARTESIAN_POINT('Origin',(12.5894081390099,-2.95236225216862,-0.999999999999996));
#11220=CARTESIAN_POINT('',(12.5976687587696,0.735143335401439,-0.999999999999996));
#11221=CARTESIAN_POINT('Origin',(12.5982736017145,1.00514265792839,-0.999999999999996));
#11222=CARTESIAN_POINT('',(12.3292713184039,0.981952755520918,-0.999999999999996));
#11223=CARTESIAN_POINT('Origin',(1.56125112837913E-14,-0.0809177714881191,
-0.999999999999996));
#11224=CARTESIAN_POINT('Origin',(12.58940813901,2.79052670919212,-0.999999999999996));
#11225=CARTESIAN_POINT('',(12.5976687587696,-0.896978878377932,-0.999999999999996));
#11226=CARTESIAN_POINT('Origin',(11.7172924887636,-5.50709943348249,-0.999999999999996));
#11227=CARTESIAN_POINT('Origin',(1.56125112837913E-14,-0.0809177714881191,
-0.999999999999996));
#11228=CARTESIAN_POINT('',(12.3292713184038,-1.14378829849741,-0.999999999999996));
#11229=CARTESIAN_POINT('Origin',(12.5982736017145,-1.16697820090488,-0.999999999999996));
#11230=CARTESIAN_POINT('Origin',(12.9113062428988,0.110293625353165,-0.999999999999996));
#11231=CARTESIAN_POINT('',(12.1527108266856,-3.49834859724242,-0.999999999999996));
#11232=CARTESIAN_POINT('Origin',(10.3330749309508,-7.82468643845875,-0.999999999999996));
#11233=CARTESIAN_POINT('Origin',(1.56125112837913E-14,-0.0809177714881191,
-0.999999999999996));
#11234=CARTESIAN_POINT('',(11.838863950502,-3.68396167373318,-0.999999999999996));
#11235=CARTESIAN_POINT('Origin',(12.0971664366947,-3.76257354069125,-0.999999999999996));
#11236=CARTESIAN_POINT('Origin',(12.6689183086518,-2.57829631406185,-0.999999999999996));
#11237=CARTESIAN_POINT('',(11.176621116299,-5.95036019036894,-0.999999999999996));
#11238=CARTESIAN_POINT('Origin',(8.49725241506067,-9.80383359396365,-0.999999999999996));
#11239=CARTESIAN_POINT('Origin',(1.56125112837913E-14,-0.0809177714881191,
-0.999999999999996));
#11240=CARTESIAN_POINT('',(10.8310414187911,-6.06666474111799,-0.999999999999996));
#11241=CARTESIAN_POINT('Origin',(11.0673550497465,-6.197262856819,-0.999999999999996));
#11242=CARTESIAN_POINT('Origin',(10.557857409218,-7.51529989933301,-0.999999999999996));
#11243=CARTESIAN_POINT('',(7.82303414640502,-9.98886158592504,-0.999999999999996));
#11244=CARTESIAN_POINT('Origin',(3.80796020367901,-12.4193872788215,-0.999999999999996));
#11245=CARTESIAN_POINT('Origin',(1.56125112837913E-14,-0.0809177714881191,
-0.999999999999996));
#11246=CARTESIAN_POINT('',(7.46002606094704,-9.95455115388547,-0.999999999999996));
#11247=CARTESIAN_POINT('Origin',(7.62279026591315,-10.1699758822287,-0.999999999999996));
#11248=CARTESIAN_POINT('Origin',(11.8728378521018,-5.15773882741456,-0.999999999999996));
#11249=CARTESIAN_POINT('',(9.71205943175165,-8.14584898508081,-0.999999999999996));
#11250=CARTESIAN_POINT('Origin',(6.2900591942915,-11.3580426722999,-0.999999999999996));
#11251=CARTESIAN_POINT('Origin',(1.56125112837913E-14,-0.0809177714881191,
-0.999999999999996));
#11252=CARTESIAN_POINT('',(9.34985040397592,-8.18776194312925,-0.999999999999996));
#11253=CARTESIAN_POINT('Origin',(9.55384714006266,-8.36463854323778,-0.999999999999996));
#11254=CARTESIAN_POINT('Origin',(8.78144793533068,-9.54794279814121,-0.999999999999996));
#11255=CARTESIAN_POINT('',(5.59210472977776,-11.3988494984891,-0.999999999999996));
#11256=CARTESIAN_POINT('Origin',(1.56125112837913E-14,-0.0809177714881191,
-0.999999999999996));
#11257=CARTESIAN_POINT('',(5.2441627818781,-11.2898152068813,-0.999999999999996));
#11258=CARTESIAN_POINT('Origin',(5.35858087893726,-11.5343729691081,-0.999999999999996));
#11259=CARTESIAN_POINT('Origin',(6.62124704860704,-11.1668312754585,-0.999999999999996));
#11260=CARTESIAN_POINT('',(3.11677350256355,-12.3141894851212,-0.999999999999996));
#11261=CARTESIAN_POINT('Origin',(1.56125112837913E-14,-0.0809177714881191,
-0.999999999999996));
#11262=CARTESIAN_POINT('',(2.79910442495613,-12.1351966556931,-0.999999999999996));
#11263=CARTESIAN_POINT('Origin',(2.8601757942279,-12.3981991040758,-0.999999999999996));
#11264=CARTESIAN_POINT('Origin',(8.78144793533087,9.3861072551648,-0.999999999999996));
#11265=CARTESIAN_POINT('',(5.59210472977799,11.2370139555127,-0.999999999999996));
#11266=CARTESIAN_POINT('Origin',(5.35858087893749,11.3725374261318,-0.999999999999996));
#11267=CARTESIAN_POINT('',(5.24416278187833,11.127979663905,-0.999999999999996));
#11268=CARTESIAN_POINT('Origin',(1.56125112837913E-14,-0.0809177714881191,
-0.999999999999996));
#11269=CARTESIAN_POINT('Origin',(6.62124704860727,11.0049957324821,-0.999999999999996));
#11270=CARTESIAN_POINT('',(3.11677350256379,12.1523539421449,-0.999999999999996));
#11271=CARTESIAN_POINT('Origin',(2.86017579422815,12.2363635610995,-0.999999999999996));
#11272=CARTESIAN_POINT('',(2.79910442495637,11.9733611127168,-0.999999999999996));
#11273=CARTESIAN_POINT('Origin',(1.56125112837913E-14,-0.0809177714881191,
-0.999999999999996));
#11274=CARTESIAN_POINT('Origin',(-4.17166589359099,12.1393765935609,-0.999999999999996));
#11275=CARTESIAN_POINT('',(-0.505224317348838,12.5330412531408,-0.999999999999996));
#11276=CARTESIAN_POINT('Origin',(4.17166589359102,12.1393765935609,-0.999999999999996));
#11277=CARTESIAN_POINT('',(0.505224317348871,12.5330412531408,-0.999999999999996));
#11278=CARTESIAN_POINT('Origin',(0.236767302664764,12.5618653969598,-0.999999999999996));
#11279=CARTESIAN_POINT('',(0.231711773070499,12.2919127314413,-0.999999999999996));
#11280=CARTESIAN_POINT('Origin',(1.56125112837913E-14,-0.0809177714881191,
-0.999999999999996));
#11281=CARTESIAN_POINT('',(-0.231711773070462,12.2919127314413,-0.999999999999996));
#11282=CARTESIAN_POINT('Origin',(-0.236767302664727,12.5618653969598,-0.999999999999996));
#11283=CARTESIAN_POINT('Origin',(-6.62124704860708,11.0049957324822,-0.999999999999996));
#11284=CARTESIAN_POINT('',(-3.11677350256359,12.1523539421449,-0.999999999999996));
#11285=CARTESIAN_POINT('Origin',(1.53976292115111,12.7396719514087,-0.999999999999996));
#11286=CARTESIAN_POINT('',(-2.12840559486928,12.3624380262694,-0.999999999999996));
#11287=CARTESIAN_POINT('Origin',(-2.39698905616047,12.3348169415543,-0.999999999999996));
#11288=CARTESIAN_POINT('',(-2.34580779517484,12.0697122857598,-0.999999999999996));
#11289=CARTESIAN_POINT('Origin',(1.56125112837913E-14,-0.0809177714881191,
-0.999999999999996));
#11290=CARTESIAN_POINT('',(-2.79910442495618,11.9733611127169,-0.999999999999996));
#11291=CARTESIAN_POINT('Origin',(-2.86017579422795,12.2363635610995,-0.999999999999996));
#11292=CARTESIAN_POINT('Origin',(-11.8728378521018,4.99590328443824,-0.999999999999996));
#11293=CARTESIAN_POINT('',(-9.71205943175167,7.98401344210451,-0.999999999999996));
#11294=CARTESIAN_POINT('Origin',(-6.29005919429154,11.1962071293236,-0.999999999999996));
#11295=CARTESIAN_POINT('',(-9.03593732412191,8.7349231163908,-0.999999999999996));
#11296=CARTESIAN_POINT('Origin',(-9.23699064246666,8.55470779189656,-0.999999999999996));
#11297=CARTESIAN_POINT('',(-9.03975952554566,8.37031721047198,-0.999999999999996));
#11298=CARTESIAN_POINT('Origin',(1.56125112837913E-14,-0.0809177714881191,
-0.999999999999996));
#11299=CARTESIAN_POINT('',(-9.34985040397594,8.02592640015294,-0.999999999999996));
#11300=CARTESIAN_POINT('Origin',(-9.55384714006268,8.20280300026147,-0.999999999999996));
#11301=CARTESIAN_POINT('Origin',(-12.6689183086518,2.41646077108552,-0.999999999999996));
#11302=CARTESIAN_POINT('',(-11.176621116299,5.78852464739263,-0.999999999999996));
#11303=CARTESIAN_POINT('Origin',(-8.49725241506071,9.64199805098735,-0.999999999999996));
#11304=CARTESIAN_POINT('',(-10.6713967989501,6.66359883426014,-0.999999999999996));
#11305=CARTESIAN_POINT('Origin',(-10.8305877470818,6.44552031162906,-0.999999999999996));
#11306=CARTESIAN_POINT('',(-10.5993296457206,6.30616576181161,-0.999999999999996));
#11307=CARTESIAN_POINT('Origin',(1.56125112837913E-14,-0.0809177714881191,
-0.999999999999996));
#11308=CARTESIAN_POINT('',(-10.8310414187911,5.90482919814167,-0.999999999999996));
#11309=CARTESIAN_POINT('Origin',(-11.0673550497465,6.03542731384268,-0.999999999999996));
#11310=CARTESIAN_POINT('Origin',(-10.557857409218,7.3534643563567,-0.999999999999996));
#11311=CARTESIAN_POINT('',(-7.82303414640506,9.82702604294875,-0.999999999999996));
#11312=CARTESIAN_POINT('Origin',(-3.80796020367907,12.2575517358453,-0.999999999999996));
#11313=CARTESIAN_POINT('',(-7.00556402899164,10.4209528486231,-0.999999999999996));
#11314=CARTESIAN_POINT('Origin',(-7.239692722777,10.2864769967152,-0.999999999999996));
#11315=CARTESIAN_POINT('',(-7.08510853652553,10.0651091368959,-0.999999999999996));
#11316=CARTESIAN_POINT('Origin',(1.56125112837913E-14,-0.0809177714881191,
-0.999999999999996));
#11317=CARTESIAN_POINT('',(-7.46002606094707,9.79271561090918,-0.999999999999996));
#11318=CARTESIAN_POINT('Origin',(-7.62279026591319,10.0081403392524,-0.999999999999996));
#11319=CARTESIAN_POINT('Origin',(-8.78144793533071,9.38610725516492,-0.999999999999996));
#11320=CARTESIAN_POINT('',(-5.5921047297778,11.2370139555128,-0.999999999999996));
#11321=CARTESIAN_POINT('Origin',(-1.15943507954543,12.7796460183509,-0.999999999999996));
#11322=CARTESIAN_POINT('',(-4.66901396936854,11.6480004411903,-0.999999999999996));
#11323=CARTESIAN_POINT('Origin',(-4.92598549120196,11.5651413018838,-0.999999999999996));
#11324=CARTESIAN_POINT('',(-4.82080430633644,11.3164710013847,-0.999999999999996));
#11325=CARTESIAN_POINT('Origin',(1.56125112837913E-14,-0.0809177714881191,
-0.999999999999996));
#11326=CARTESIAN_POINT('',(-5.24416278187814,11.1279796639051,-0.999999999999996));
#11327=CARTESIAN_POINT('Origin',(-5.3585808789373,11.3725374261318,-0.999999999999996));
#11328=CARTESIAN_POINT('Origin',(-12.9113062428988,-0.272129168329486,-0.999999999999996));
#11329=CARTESIAN_POINT('',(-12.1527108266856,3.3365130542661,-0.999999999999996));
#11330=CARTESIAN_POINT('Origin',(-10.3330749309508,7.66285089548245,-0.999999999999996));
#11331=CARTESIAN_POINT('',(-11.8404650266211,4.29750681267689,-0.999999999999996));
#11332=CARTESIAN_POINT('Origin',(-11.9508361962233,4.0510961698048,-0.999999999999996));
#11333=CARTESIAN_POINT('',(-11.6956581991509,3.96286811411883,-0.999999999999996));
#11334=CARTESIAN_POINT('Origin',(1.56125112837913E-14,-0.0809177714881191,
-0.999999999999996));
#11335=CARTESIAN_POINT('',(-11.838863950502,3.52212613075686,-0.999999999999996));
#11336=CARTESIAN_POINT('Origin',(-12.0971664366947,3.60073799771494,-0.999999999999996));
#11337=CARTESIAN_POINT('Origin',(-12.5894081390099,-2.95236225216845,-0.999999999999996));
#11338=CARTESIAN_POINT('',(-12.5976687587696,0.73514333540161,-0.999999999999996));
#11339=CARTESIAN_POINT('Origin',(-11.7172924887636,5.34526389050617,-0.999999999999996));
#11340=CARTESIAN_POINT('',(-12.4920481157737,1.74005662675346,-0.999999999999996));
#11341=CARTESIAN_POINT('Origin',(-12.5487757571153,1.47608319114332,-0.999999999999996));
#11342=CARTESIAN_POINT('',(-12.2808303672836,1.44283761898748,-0.999999999999996));
#11343=CARTESIAN_POINT('Origin',(1.56125112837913E-14,-0.0809177714881191,
-0.999999999999996));
#11344=CARTESIAN_POINT('',(-12.3292713184038,0.981952755521089,-0.999999999999996));
#11345=CARTESIAN_POINT('Origin',(-12.5982736017144,1.00514265792856,-0.999999999999996));
#11346=CARTESIAN_POINT('Origin',(-11.7172924887636,-5.50709943348233,-0.999999999999996));
#11347=CARTESIAN_POINT('',(-12.4920481157737,-1.90189216972961,-0.999999999999996));
#11348=CARTESIAN_POINT('Origin',(-12.5894081390099,2.79052670919229,-0.999999999999996));
#11349=CARTESIAN_POINT('',(-12.5976687587696,-0.896978878377764,-0.999999999999996));
#11350=CARTESIAN_POINT('Origin',(-12.5982736017144,-1.16697820090471,-0.999999999999996));
#11351=CARTESIAN_POINT('',(-12.3292713184038,-1.14378829849724,-0.999999999999996));
#11352=CARTESIAN_POINT('Origin',(1.56125112837913E-14,-0.0809177714881191,
-0.999999999999996));
#11353=CARTESIAN_POINT('',(-12.2808303672837,-1.60467316196364,-0.999999999999996));
#11354=CARTESIAN_POINT('Origin',(-12.5487757571153,-1.63791873411947,-0.999999999999996));
#11355=CARTESIAN_POINT('Origin',(-10.3330749309508,-7.82468643845862,-0.999999999999996));
#11356=CARTESIAN_POINT('',(-11.8404650266211,-4.45934235565305,-0.999999999999996));
#11357=CARTESIAN_POINT('Origin',(-12.9113062428988,0.110293625353334,-0.999999999999996));
#11358=CARTESIAN_POINT('',(-12.1527108266856,-3.49834859724226,-0.999999999999996));
#11359=CARTESIAN_POINT('Origin',(-12.0971664366948,-3.76257354069109,-0.999999999999996));
#11360=CARTESIAN_POINT('',(-11.838863950502,-3.68396167373302,-0.999999999999996));
#11361=CARTESIAN_POINT('Origin',(1.56125112837913E-14,-0.0809177714881191,
-0.999999999999996));
#11362=CARTESIAN_POINT('',(-11.6956581991509,-4.12470365709499,-0.999999999999996));
#11363=CARTESIAN_POINT('Origin',(-11.9508361962233,-4.21293171278096,-0.999999999999996));
#11364=CARTESIAN_POINT('Origin',(-1.15943507954552,-12.9414815613271,-0.999999999999996));
#11365=CARTESIAN_POINT('',(-4.66901396936862,-11.8098359841665,-0.999999999999996));
#11366=CARTESIAN_POINT('Origin',(-8.78144793533077,-9.5479427981411,-0.999999999999996));
#11367=CARTESIAN_POINT('',(-5.59210472977788,-11.398849498489,-0.999999999999996));
#11368=CARTESIAN_POINT('Origin',(-5.35858087893738,-11.534372969108,-0.999999999999996));
#11369=CARTESIAN_POINT('',(-5.24416278187822,-11.2898152068813,-0.999999999999996));
#11370=CARTESIAN_POINT('Origin',(1.56125112837913E-14,-0.0809177714881191,
-0.999999999999996));
#11371=CARTESIAN_POINT('',(-4.82080430633652,-11.4783065443609,-0.999999999999996));
#11372=CARTESIAN_POINT('Origin',(-4.92598549120204,-11.72697684486,-0.999999999999996));
#11373=CARTESIAN_POINT('Origin',(-3.80796020367915,-12.4193872788215,-0.999999999999996));
#11374=CARTESIAN_POINT('',(-7.00556402899171,-10.5827883915993,-0.999999999999996));
#11375=CARTESIAN_POINT('Origin',(-10.5578574092181,-7.51529989933287,-0.999999999999996));
#11376=CARTESIAN_POINT('',(-7.82303414640512,-9.98886158592494,-0.999999999999996));
#11377=CARTESIAN_POINT('Origin',(-7.62279026591326,-10.1699758822286,-0.999999999999996));
#11378=CARTESIAN_POINT('',(-7.46002606094714,-9.95455115388536,-0.999999999999996));
#11379=CARTESIAN_POINT('Origin',(1.56125112837913E-14,-0.0809177714881191,
-0.999999999999996));
#11380=CARTESIAN_POINT('',(-7.0851085365256,-10.2269446798721,-0.999999999999996));
#11381=CARTESIAN_POINT('Origin',(-7.23969272277707,-10.4483125396914,-0.999999999999996));
#11382=CARTESIAN_POINT('Origin',(-8.49725241506077,-9.80383359396353,-0.999999999999996));
#11383=CARTESIAN_POINT('',(-10.6713967989502,-6.82543437723631,-0.999999999999996));
#11384=CARTESIAN_POINT('Origin',(-12.6689183086518,-2.57829631406167,-0.999999999999996));
#11385=CARTESIAN_POINT('',(-11.176621116299,-5.95036019036879,-0.999999999999996));
#11386=CARTESIAN_POINT('Origin',(-11.0673550497465,-6.19726285681884,-0.999999999999996));
#11387=CARTESIAN_POINT('',(-10.8310414187911,-6.06666474111783,-0.999999999999996));
#11388=CARTESIAN_POINT('Origin',(1.56125112837913E-14,-0.0809177714881191,
-0.999999999999996));
#11389=CARTESIAN_POINT('',(-10.5993296457206,-6.46800130478777,-0.999999999999996));
#11390=CARTESIAN_POINT('Origin',(-10.8305877470818,-6.60735585460522,-0.999999999999996));
#11391=CARTESIAN_POINT('Origin',(-6.29005919429162,-11.3580426722998,-0.999999999999996));
#11392=CARTESIAN_POINT('',(-9.03593732412197,-8.89675865936698,-0.999999999999996));
#11393=CARTESIAN_POINT('Origin',(-11.8728378521018,-5.1577388274144,-0.999999999999996));
#11394=CARTESIAN_POINT('',(-9.71205943175173,-8.14584898508068,-0.999999999999996));
#11395=CARTESIAN_POINT('Origin',(-9.55384714006274,-8.36463854323765,-0.999999999999996));
#11396=CARTESIAN_POINT('',(-9.349850403976,-8.18776194312912,-0.999999999999996));
#11397=CARTESIAN_POINT('Origin',(1.56125112837913E-14,-0.0809177714881191,
-0.999999999999996));
#11398=CARTESIAN_POINT('',(-9.03975952554573,-8.53215275344816,-0.999999999999996));
#11399=CARTESIAN_POINT('Origin',(-9.23699064246672,-8.71654333487274,-0.999999999999996));
#11400=CARTESIAN_POINT('Origin',(-0.749999999999984,3.66908222851188,-0.999999999999996));
#11401=CARTESIAN_POINT('',(-0.749999999999984,3.66908222851188,-0.999999999999996));
#11402=CARTESIAN_POINT('Origin',(-0.749999999999984,3.66908222851188,-0.999999999999996));
#11403=CARTESIAN_POINT('',(0.750000000000016,3.66908222851188,-0.999999999999996));
#11404=CARTESIAN_POINT('Origin',(0.750000000000016,3.66908222851188,-0.999999999999996));
#11916=UNCERTAINTY_MEASURE_WITH_UNIT(LENGTH_MEASURE(0.01),#11934,
'DISTANCE_ACCURACY_VALUE',
'Maximum model space distance between geometric entities at asserted c
onnectivities');
#11922=UNCERTAINTY_MEASURE_WITH_UNIT(LENGTH_MEASURE(0.01),#11934,
'DISTANCE_ACCURACY_VALUE',
'Maximum model space distance between geometric entities at asserted c
onnectivities');
#11927=(
GEOMETRIC_REPRESENTATION_CONTEXT(3)
GLOBAL_UNCERTAINTY_ASSIGNED_CONTEXT((#11916))
GLOBAL_UNIT_ASSIGNED_CONTEXT((#11934,#11936,#11937))
REPRESENTATION_CONTEXT('','3D')
);
#11933=(
GEOMETRIC_REPRESENTATION_CONTEXT(3)
GLOBAL_UNCERTAINTY_ASSIGNED_CONTEXT((#11922))
GLOBAL_UNIT_ASSIGNED_CONTEXT((#11934,#11936,#11937))
REPRESENTATION_CONTEXT('','3D')
);
#11934=(
LENGTH_UNIT()
NAMED_UNIT(*)
SI_UNIT(.MILLI.,.METRE.)
);
#11936=(
NAMED_UNIT(*)
PLANE_ANGLE_UNIT()
SI_UNIT($,.RADIAN.)
);
#11937=(
NAMED_UNIT(*)
SI_UNIT($,.STERADIAN.)
SOLID_ANGLE_UNIT()
);
#11942=SHAPE_DEFINITION_REPRESENTATION(#11952,#11991);
#11952=PRODUCT_DEFINITION_SHAPE('',$,#12002);
#11991=SHAPE_REPRESENTATION('',(#6899),#11927);
#11997=PRODUCT_DEFINITION_CONTEXT('part definition',#12029,'design');
#12002=PRODUCT_DEFINITION('Spur Gear','Spur Gear',#12012,#11997);
#12012=PRODUCT_DEFINITION_FORMATION('',$,#12035);
#12029=APPLICATION_CONTEXT(
'Core Data for Automotive Mechanical Design Process');
#12030=PRODUCT_CONTEXT('part definition',#12029,'mechanical');
#12035=PRODUCT('Spur Gear','Spur Gear',$,(#12030));
#12043=PRESENTATION_STYLE_ASSIGNMENT((#12047));
#12047=SURFACE_STYLE_USAGE(.BOTH.,#12051);
#12051=SURFACE_SIDE_STYLE('',(#12055));
#12055=SURFACE_STYLE_FILL_AREA(#12059);
#12059=FILL_AREA_STYLE('Opaque(61,176,222)',(#12063));
#12063=FILL_AREA_STYLE_COLOUR('Opaque(61,176,222)',#12067);
#12067=COLOUR_RGB('Opaque(61,176,222)',0.23921568627451,0.690196078431373,
0.870588235294118);
ENDSEC;
END-ISO-10303-21;
